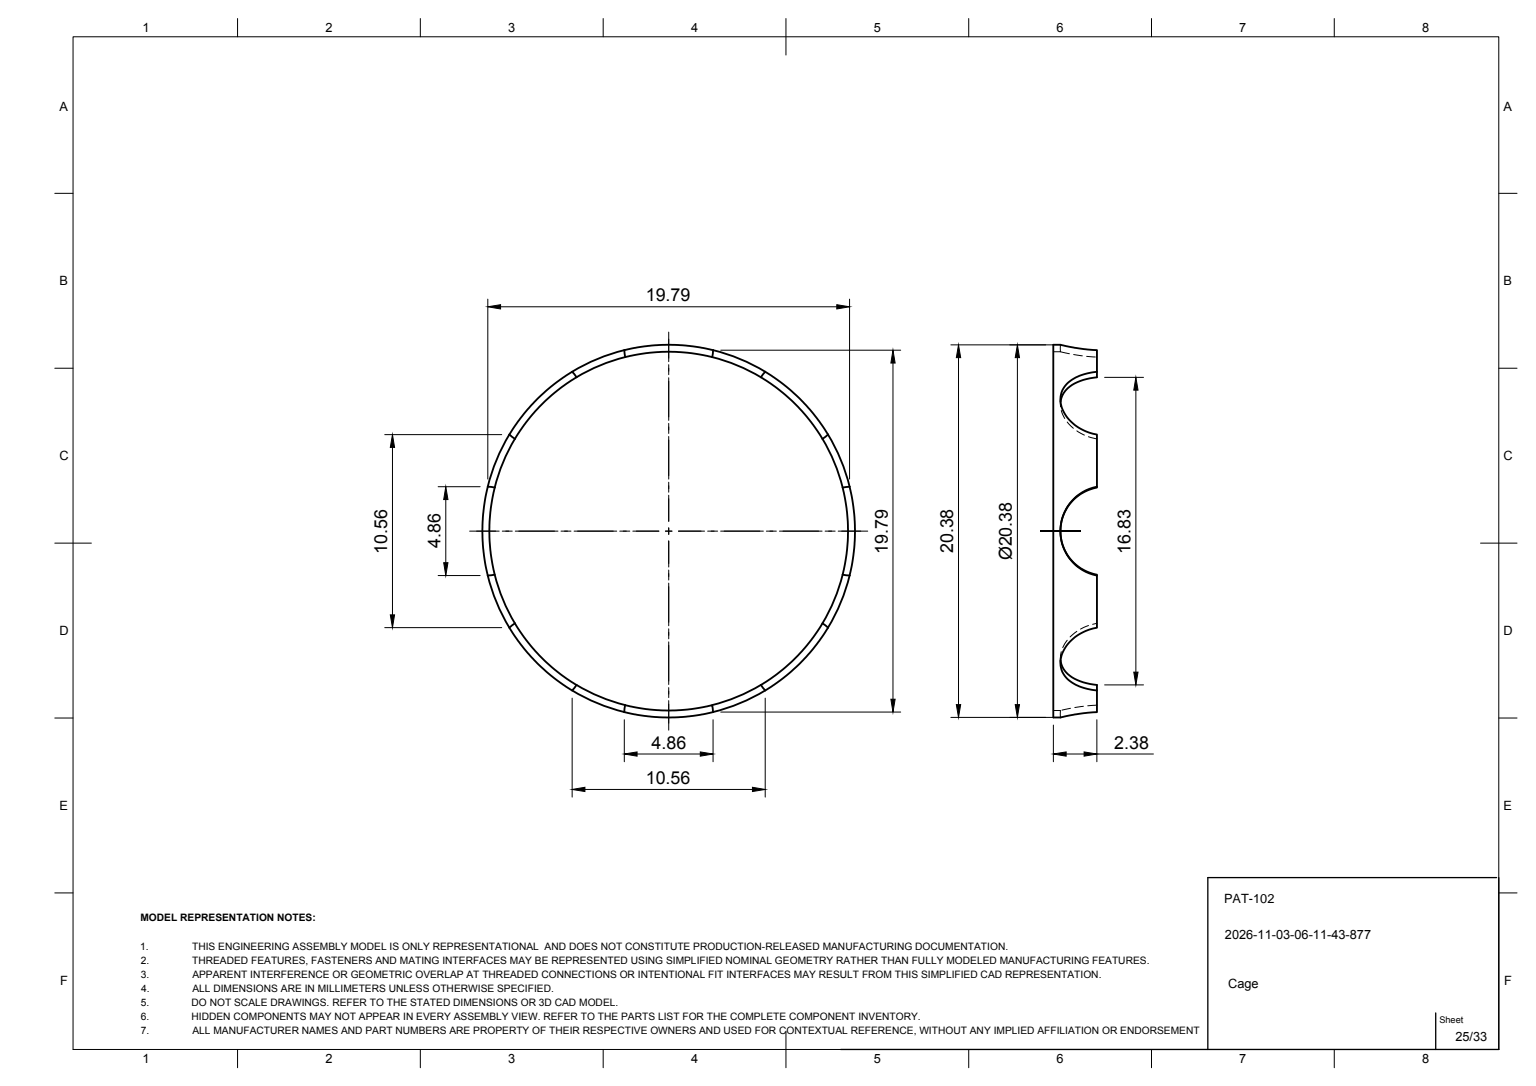
ISO-10303-21;
HEADER;
/* Generated by software containing ST-Developer
 * from STEP Tools, Inc. (www.steptools.com) 
 */

FILE_DESCRIPTION(
/* description */ ('Swing-away clamp arm'),
/* implementation_level */ '2;1');

FILE_NAME(
/* name */ 'Cage.step',
/* time_stamp */ '2026-10-28T03:26:03-07:00',
/* author */ (''),
/* organization */ (''),
/* preprocessor_version */ 'ST-DEVELOPER v20.2',
/* originating_system */ 'Autodesk Translation Framework v15.17.0.0',
/* authorisation */ '');

FILE_SCHEMA (('AUTOMOTIVE_DESIGN { 1 0 10303 214 3 1 1 }'));
ENDSEC;

DATA;
#10=MECHANICAL_DESIGN_GEOMETRIC_PRESENTATION_REPRESENTATION('',(#317),#10627);
#19=SPHERICAL_SURFACE('',#5638,0.247676);
#20=SPHERICAL_SURFACE('',#5654,0.247676);
#21=SPHERICAL_SURFACE('',#5659,0.247676);
#22=SPHERICAL_SURFACE('',#5664,0.247676);
#23=SPHERICAL_SURFACE('',#5669,0.247676);
#24=SPHERICAL_SURFACE('',#5674,0.247676);
#25=SPHERICAL_SURFACE('',#5679,0.247676);
#26=SPHERICAL_SURFACE('',#5687,0.247676);
#222=B_SPLINE_CURVE_WITH_KNOTS('',3,(#9779,#9780,#9781,#9782,#9783,#9784,
#9785,#9786,#9787,#9788,#9789,#9790,#9791,#9792,#9793,#9794,#9795,#9796,
#9797,#9798,#9799,#9800),.UNSPECIFIED.,.F.,.F.,(4,2,2,2,2,2,2,2,2,2,4),
(0.0473477652366656,0.126350602536658,0.189525903804987,0.252701205073317,
0.313298422430275,0.373895639787233,0.434492857144191,0.495090074501149,
0.558265375769478,0.621440677037807,0.7004435143378),.UNSPECIFIED.);
#223=B_SPLINE_CURVE_WITH_KNOTS('',3,(#9804,#9805,#9806,#9807,#9808,#9809,
#9810,#9811,#9812,#9813,#9814,#9815,#9816,#9817,#9818,#9819,#9820,#9821,
#9822,#9823,#9824,#9825),.UNSPECIFIED.,.F.,.F.,(4,2,2,2,2,2,2,2,2,2,4),
(0.0464897534940957,0.0852567806515119,0.170513561303024,0.246687263103517,
0.308657850341199,0.370628437578881,0.432599024816563,0.494569612054245,
0.570743313854739,0.656000094506251,0.694767121663666),.UNSPECIFIED.);
#224=B_SPLINE_CURVE_WITH_KNOTS('',3,(#9831,#9832,#9833,#9834,#9835,#9836,
#9837,#9838,#9839,#9840,#9841,#9842,#9843,#9844,#9845,#9846,#9847,#9848,
#9849,#9850,#9851,#9852),.UNSPECIFIED.,.F.,.F.,(4,2,2,2,2,2,2,2,2,2,4),
(0.0464897534940957,0.0852567806515118,0.170513561303024,0.246687263103517,
0.308657850341199,0.370628437578881,0.432599024816563,0.494569612054245,
0.570743313854738,0.65600009450625,0.694767121663666),.UNSPECIFIED.);
#225=B_SPLINE_CURVE_WITH_KNOTS('',3,(#9856,#9857,#9858,#9859,#9860,#9861,
#9862,#9863,#9864,#9865,#9866,#9867,#9868,#9869,#9870,#9871,#9872,#9873,
#9874,#9875,#9876,#9877),.UNSPECIFIED.,.F.,.F.,(4,2,2,2,2,2,2,2,2,2,4),
(0.0464897534940957,0.0852567806515119,0.170513561303024,0.246687263103517,
0.308657850341199,0.370628437578881,0.432599024816563,0.494569612054245,
0.570743313854739,0.656000094506251,0.694767121663666),.UNSPECIFIED.);
#226=B_SPLINE_CURVE_WITH_KNOTS('',3,(#9881,#9882,#9883,#9884,#9885,#9886,
#9887,#9888,#9889,#9890,#9891,#9892),.UNSPECIFIED.,.F.,.F.,(4,2,2,2,2,4),
(0.0464897534940957,0.0852567806515119,0.170513561303024,0.246687263103517,
0.308657850341199,0.370628437578881),.UNSPECIFIED.);
#227=B_SPLINE_CURVE_WITH_KNOTS('',3,(#9897,#9898,#9899,#9900,#9901,#9902,
#9903,#9904,#9905,#9906,#9907,#9908),.UNSPECIFIED.,.F.,.F.,(4,2,2,2,2,4),
(0.370628437578881,0.432599024816563,0.494569612054245,0.570743313854738,
0.65600009450625,0.694767121663666),.UNSPECIFIED.);
#228=B_SPLINE_CURVE_WITH_KNOTS('',3,(#9912,#9913,#9914,#9915,#9916,#9917,
#9918,#9919,#9920,#9921,#9922,#9923,#9924,#9925,#9926,#9927,#9928,#9929,
#9930,#9931,#9932,#9933),.UNSPECIFIED.,.F.,.F.,(4,2,2,2,2,2,2,2,2,2,4),
(0.0464897534940957,0.0852567806515121,0.170513561303024,0.246687263103518,
0.308657850341199,0.370628437578881,0.432599024816563,0.494569612054245,
0.570743313854738,0.65600009450625,0.694767121663666),.UNSPECIFIED.);
#229=B_SPLINE_CURVE_WITH_KNOTS('',3,(#9937,#9938,#9939,#9940,#9941,#9942,
#9943,#9944,#9945,#9946,#9947,#9948,#9949,#9950,#9951,#9952,#9953,#9954,
#9955,#9956,#9957,#9958),.UNSPECIFIED.,.F.,.F.,(4,2,2,2,2,2,2,2,2,2,4),
(0.0464897534940957,0.0852567806515119,0.170513561303024,0.246687263103517,
0.308657850341199,0.370628437578881,0.432599024816563,0.494569612054245,
0.570743313854738,0.65600009450625,0.694767121663667),.UNSPECIFIED.);
#230=B_SPLINE_CURVE_WITH_KNOTS('',3,(#9962,#9963,#9964,#9965,#9966,#9967,
#9968,#9969,#9970,#9971,#9972,#9973,#9974,#9975,#9976,#9977,#9978,#9979,
#9980,#9981,#9982,#9983),.UNSPECIFIED.,.F.,.F.,(4,2,2,2,2,2,2,2,2,2,4),
(0.0464897534940957,0.0852567806515119,0.170513561303024,0.246687263103517,
0.308657850341199,0.370628437578881,0.432599024816563,0.494569612054245,
0.570743313854738,0.65600009450625,0.694767121663666),.UNSPECIFIED.);
#231=B_SPLINE_CURVE_WITH_KNOTS('',3,(#9987,#9988,#9989,#9990,#9991,#9992,
#9993,#9994,#9995,#9996,#9997,#9998,#9999,#10000,#10001,#10002,#10003,#10004,
#10005,#10006,#10007,#10008),.UNSPECIFIED.,.F.,.F.,(4,2,2,2,2,2,2,2,2,2,
4),(0.0464897534940957,0.0852567806515119,0.170513561303024,0.246687263103517,
0.308657850341199,0.370628437578881,0.432599024816563,0.494569612054245,
0.570743313854739,0.656000094506251,0.694767121663667),.UNSPECIFIED.);
#232=B_SPLINE_CURVE_WITH_KNOTS('',3,(#10016,#10017,#10018,#10019,#10020,
#10021,#10022,#10023,#10024,#10025,#10026,#10027,#10028,#10029,#10030,#10031,
#10032,#10033,#10034,#10035,#10036,#10037),.UNSPECIFIED.,.F.,.F.,(4,2,2,
2,2,2,2,2,2,2,4),(0.0473477652366656,0.126350602536658,0.189525903804987,
0.252701205073316,0.313298422430274,0.373895639787232,0.434492857144191,
0.495090074501149,0.558265375769478,0.621440677037807,0.7004435143378),
 .UNSPECIFIED.);
#233=B_SPLINE_CURVE_WITH_KNOTS('',3,(#10045,#10046,#10047,#10048,#10049,
#10050,#10051,#10052,#10053,#10054,#10055,#10056,#10057,#10058,#10059,#10060,
#10061,#10062,#10063,#10064,#10065,#10066),.UNSPECIFIED.,.F.,.F.,(4,2,2,
2,2,2,2,2,2,2,4),(0.0473477652366656,0.126350602536658,0.189525903804987,
0.252701205073317,0.313298422430275,0.373895639787233,0.434492857144191,
0.495090074501149,0.558265375769478,0.621440677037807,0.7004435143378),
 .UNSPECIFIED.);
#234=B_SPLINE_CURVE_WITH_KNOTS('',3,(#10075,#10076,#10077,#10078,#10079,
#10080,#10081,#10082,#10083,#10084,#10085,#10086),.UNSPECIFIED.,.F.,.F.,
(4,2,2,2,2,4),(0.0473477652366656,0.126350602536658,0.189525903804987,0.252701205073316,
0.313298422430275,0.373895639787233),.UNSPECIFIED.);
#235=B_SPLINE_CURVE_WITH_KNOTS('',3,(#10088,#10089,#10090,#10091,#10092,
#10093,#10094,#10095,#10096,#10097,#10098,#10099),.UNSPECIFIED.,.F.,.F.,
(4,2,2,2,2,4),(0.373895639787233,0.434492857144191,0.495090074501149,0.558265375769478,
0.621440677037807,0.7004435143378),.UNSPECIFIED.);
#236=B_SPLINE_CURVE_WITH_KNOTS('',3,(#10106,#10107,#10108,#10109,#10110,
#10111,#10112,#10113,#10114,#10115,#10116,#10117,#10118,#10119,#10120,#10121,
#10122,#10123,#10124,#10125,#10126,#10127),.UNSPECIFIED.,.F.,.F.,(4,2,2,
2,2,2,2,2,2,2,4),(0.0473477652366656,0.126350602536658,0.189525903804987,
0.252701205073316,0.313298422430275,0.373895639787233,0.434492857144191,
0.495090074501149,0.558265375769478,0.621440677037807,0.7004435143378),
 .UNSPECIFIED.);
#237=B_SPLINE_CURVE_WITH_KNOTS('',3,(#10135,#10136,#10137,#10138,#10139,
#10140,#10141,#10142,#10143,#10144,#10145,#10146,#10147,#10148,#10149,#10150,
#10151,#10152,#10153,#10154,#10155,#10156),.UNSPECIFIED.,.F.,.F.,(4,2,2,
2,2,2,2,2,2,2,4),(0.0473477652366656,0.126350602536658,0.189525903804987,
0.252701205073317,0.313298422430275,0.373895639787233,0.434492857144191,
0.495090074501149,0.558265375769478,0.621440677037807,0.7004435143378),
 .UNSPECIFIED.);
#238=B_SPLINE_CURVE_WITH_KNOTS('',3,(#10164,#10165,#10166,#10167,#10168,
#10169,#10170,#10171,#10172,#10173,#10174,#10175,#10176,#10177,#10178,#10179,
#10180,#10181,#10182,#10183,#10184,#10185),.UNSPECIFIED.,.F.,.F.,(4,2,2,
2,2,2,2,2,2,2,4),(0.0473477652366656,0.126350602536658,0.189525903804987,
0.252701205073316,0.313298422430275,0.373895639787233,0.434492857144191,
0.495090074501149,0.558265375769478,0.621440677037807,0.7004435143378),
 .UNSPECIFIED.);
#239=B_SPLINE_CURVE_WITH_KNOTS('',3,(#10194,#10195,#10196,#10197,#10198,
#10199,#10200,#10201,#10202,#10203,#10204,#10205,#10206,#10207,#10208,#10209,
#10210,#10211,#10212,#10213,#10214,#10215),.UNSPECIFIED.,.F.,.F.,(4,2,2,
2,2,2,2,2,2,2,4),(0.0473477652366656,0.126350602536658,0.189525903804987,
0.252701205073317,0.313298422430275,0.373895639787233,0.434492857144191,
0.495090074501149,0.558265375769478,0.621440677037807,0.7004435143378),
 .UNSPECIFIED.);
#258=SHAPE_REPRESENTATION_RELATIONSHIP('SRR','None',#10758,#284);
#284=ADVANCED_BREP_SHAPE_REPRESENTATION('',(#350),#10617);
#317=STYLED_ITEM('',(#10965),#350);
#350=MANIFOLD_SOLID_BREP('Continuous crown cage',#4924);
#436=FACE_BOUND('',#1250,.T.);
#582=PLANE('',#5651);
#583=PLANE('',#5656);
#584=PLANE('',#5661);
#585=PLANE('',#5666);
#586=PLANE('',#5671);
#587=PLANE('',#5676);
#588=PLANE('',#5685);
#589=PLANE('',#5689);
#590=PLANE('',#5690);
#847=FACE_OUTER_BOUND('',#1232,.T.);
#848=FACE_OUTER_BOUND('',#1233,.T.);
#849=FACE_OUTER_BOUND('',#1234,.T.);
#850=FACE_OUTER_BOUND('',#1235,.T.);
#851=FACE_OUTER_BOUND('',#1236,.T.);
#852=FACE_OUTER_BOUND('',#1237,.T.);
#853=FACE_OUTER_BOUND('',#1238,.T.);
#854=FACE_OUTER_BOUND('',#1239,.T.);
#855=FACE_OUTER_BOUND('',#1240,.T.);
#856=FACE_OUTER_BOUND('',#1241,.T.);
#857=FACE_OUTER_BOUND('',#1242,.T.);
#858=FACE_OUTER_BOUND('',#1243,.T.);
#859=FACE_OUTER_BOUND('',#1244,.T.);
#860=FACE_OUTER_BOUND('',#1245,.T.);
#861=FACE_OUTER_BOUND('',#1246,.T.);
#862=FACE_OUTER_BOUND('',#1247,.T.);
#863=FACE_OUTER_BOUND('',#1248,.T.);
#864=FACE_OUTER_BOUND('',#1249,.T.);
#865=FACE_OUTER_BOUND('',#1251,.T.);
#1232=EDGE_LOOP('',(#4121,#4122,#4123,#4124));
#1233=EDGE_LOOP('',(#4125,#4126,#4127,#4128,#4129,#4130,#4131,#4132,#4133,
#4134,#4135,#4136,#4137,#4138,#4139,#4140,#4141,#4142,#4143,#4144));
#1234=EDGE_LOOP('',(#4145,#4146,#4147,#4148));
#1235=EDGE_LOOP('',(#4149,#4150,#4151,#4152));
#1236=EDGE_LOOP('',(#4153,#4154,#4155,#4156));
#1237=EDGE_LOOP('',(#4157,#4158,#4159,#4160));
#1238=EDGE_LOOP('',(#4161,#4162,#4163,#4164));
#1239=EDGE_LOOP('',(#4165,#4166,#4167,#4168,#4169,#4170));
#1240=EDGE_LOOP('',(#4171,#4172,#4173,#4174));
#1241=EDGE_LOOP('',(#4175,#4176,#4177,#4178));
#1242=EDGE_LOOP('',(#4179,#4180,#4181,#4182));
#1243=EDGE_LOOP('',(#4183,#4184,#4185,#4186));
#1244=EDGE_LOOP('',(#4187,#4188,#4189,#4190));
#1245=EDGE_LOOP('',(#4191,#4192,#4193,#4194));
#1246=EDGE_LOOP('',(#4195,#4196,#4197,#4198,#4199,#4200,#4201,#4202,#4203,
#4204,#4205,#4206,#4207,#4208,#4209,#4210,#4211,#4212,#4213,#4214));
#1247=EDGE_LOOP('',(#4215,#4216,#4217,#4218));
#1248=EDGE_LOOP('',(#4219,#4220,#4221,#4222));
#1249=EDGE_LOOP('',(#4223));
#1250=EDGE_LOOP('',(#4224));
#1251=EDGE_LOOP('',(#4225,#4226,#4227,#4228));
#1596=LINE('',#9894,#1918);
#1597=LINE('',#10190,#1919);
#1918=VECTOR('',#6959,1.019052);
#1919=VECTOR('',#7036,0.980948);
#2169=CIRCLE('',#5639,0.243053047864041);
#2170=CIRCLE('',#5640,0.243053047864041);
#2171=CIRCLE('',#5642,1.019052);
#2172=CIRCLE('',#5643,1.019052);
#2173=CIRCLE('',#5644,1.019052);
#2174=CIRCLE('',#5645,1.019052);
#2175=CIRCLE('',#5646,1.019052);
#2176=CIRCLE('',#5647,1.019052);
#2177=CIRCLE('',#5648,1.019052);
#2178=CIRCLE('',#5649,1.019052);
#2179=CIRCLE('',#5650,1.019052);
#2180=CIRCLE('',#5652,0.980948);
#2181=CIRCLE('',#5653,0.243053047864041);
#2182=CIRCLE('',#5655,0.243053047864041);
#2183=CIRCLE('',#5657,0.980948);
#2184=CIRCLE('',#5658,0.243053047864041);
#2185=CIRCLE('',#5660,0.243053047864041);
#2186=CIRCLE('',#5662,0.980948);
#2187=CIRCLE('',#5663,0.243053047864041);
#2188=CIRCLE('',#5665,0.243053047864041);
#2189=CIRCLE('',#5667,0.980948);
#2190=CIRCLE('',#5668,0.243053047864041);
#2191=CIRCLE('',#5670,0.243053047864041);
#2192=CIRCLE('',#5672,0.980948);
#2193=CIRCLE('',#5673,0.243053047864041);
#2194=CIRCLE('',#5675,0.243053047864041);
#2195=CIRCLE('',#5677,0.980948);
#2196=CIRCLE('',#5678,0.243053047864041);
#2197=CIRCLE('',#5680,0.243053047864041);
#2198=CIRCLE('',#5682,0.980948);
#2199=CIRCLE('',#5683,0.980948);
#2200=CIRCLE('',#5684,0.980948);
#2201=CIRCLE('',#5686,0.243053047864041);
#2202=CIRCLE('',#5688,0.243053047864041);
#2550=VERTEX_POINT('',#9777);
#2551=VERTEX_POINT('',#9778);
#2552=VERTEX_POINT('',#9801);
#2553=VERTEX_POINT('',#9803);
#2554=VERTEX_POINT('',#9828);
#2555=VERTEX_POINT('',#9830);
#2556=VERTEX_POINT('',#9853);
#2557=VERTEX_POINT('',#9855);
#2558=VERTEX_POINT('',#9878);
#2559=VERTEX_POINT('',#9880);
#2560=VERTEX_POINT('',#9893);
#2561=VERTEX_POINT('',#9896);
#2562=VERTEX_POINT('',#9909);
#2563=VERTEX_POINT('',#9911);
#2564=VERTEX_POINT('',#9934);
#2565=VERTEX_POINT('',#9936);
#2566=VERTEX_POINT('',#9959);
#2567=VERTEX_POINT('',#9961);
#2568=VERTEX_POINT('',#9984);
#2569=VERTEX_POINT('',#9986);
#2570=VERTEX_POINT('',#10011);
#2571=VERTEX_POINT('',#10015);
#2572=VERTEX_POINT('',#10040);
#2573=VERTEX_POINT('',#10044);
#2574=VERTEX_POINT('',#10069);
#2575=VERTEX_POINT('',#10073);
#2576=VERTEX_POINT('',#10074);
#2577=VERTEX_POINT('',#10101);
#2578=VERTEX_POINT('',#10105);
#2579=VERTEX_POINT('',#10130);
#2580=VERTEX_POINT('',#10134);
#2581=VERTEX_POINT('',#10159);
#2582=VERTEX_POINT('',#10163);
#2583=VERTEX_POINT('',#10188);
#2584=VERTEX_POINT('',#10191);
#2585=VERTEX_POINT('',#10193);
#3093=EDGE_CURVE('',#2550,#2551,#222,.T.);
#3094=EDGE_CURVE('',#2552,#2550,#2169,.T.);
#3095=EDGE_CURVE('',#2553,#2552,#223,.T.);
#3096=EDGE_CURVE('',#2551,#2553,#2170,.T.);
#3097=EDGE_CURVE('',#2554,#2552,#2171,.T.);
#3098=EDGE_CURVE('',#2554,#2555,#224,.T.);
#3099=EDGE_CURVE('',#2556,#2555,#2172,.T.);
#3100=EDGE_CURVE('',#2556,#2557,#225,.T.);
#3101=EDGE_CURVE('',#2558,#2557,#2173,.T.);
#3102=EDGE_CURVE('',#2558,#2559,#226,.T.);
#3103=EDGE_CURVE('',#2559,#2560,#1596,.T.);
#3104=EDGE_CURVE('',#2560,#2560,#2174,.T.);
#3105=EDGE_CURVE('',#2559,#2561,#227,.T.);
#3106=EDGE_CURVE('',#2562,#2561,#2175,.T.);
#3107=EDGE_CURVE('',#2562,#2563,#228,.T.);
#3108=EDGE_CURVE('',#2564,#2563,#2176,.T.);
#3109=EDGE_CURVE('',#2564,#2565,#229,.T.);
#3110=EDGE_CURVE('',#2566,#2565,#2177,.T.);
#3111=EDGE_CURVE('',#2566,#2567,#230,.T.);
#3112=EDGE_CURVE('',#2568,#2567,#2178,.T.);
#3113=EDGE_CURVE('',#2568,#2569,#231,.T.);
#3114=EDGE_CURVE('',#2553,#2569,#2179,.T.);
#3115=EDGE_CURVE('',#2550,#2570,#2180,.T.);
#3116=EDGE_CURVE('',#2570,#2554,#2181,.T.);
#3117=EDGE_CURVE('',#2571,#2570,#232,.T.);
#3118=EDGE_CURVE('',#2555,#2571,#2182,.T.);
#3119=EDGE_CURVE('',#2571,#2572,#2183,.T.);
#3120=EDGE_CURVE('',#2572,#2556,#2184,.T.);
#3121=EDGE_CURVE('',#2573,#2572,#233,.T.);
#3122=EDGE_CURVE('',#2557,#2573,#2185,.T.);
#3123=EDGE_CURVE('',#2573,#2574,#2186,.T.);
#3124=EDGE_CURVE('',#2574,#2558,#2187,.T.);
#3125=EDGE_CURVE('',#2575,#2576,#234,.T.);
#3126=EDGE_CURVE('',#2561,#2575,#2188,.T.);
#3127=EDGE_CURVE('',#2576,#2574,#235,.T.);
#3128=EDGE_CURVE('',#2575,#2577,#2189,.T.);
#3129=EDGE_CURVE('',#2577,#2562,#2190,.T.);
#3130=EDGE_CURVE('',#2578,#2577,#236,.T.);
#3131=EDGE_CURVE('',#2563,#2578,#2191,.T.);
#3132=EDGE_CURVE('',#2578,#2579,#2192,.T.);
#3133=EDGE_CURVE('',#2579,#2564,#2193,.T.);
#3134=EDGE_CURVE('',#2580,#2579,#237,.T.);
#3135=EDGE_CURVE('',#2565,#2580,#2194,.T.);
#3136=EDGE_CURVE('',#2580,#2581,#2195,.T.);
#3137=EDGE_CURVE('',#2581,#2566,#2196,.T.);
#3138=EDGE_CURVE('',#2582,#2581,#238,.T.);
#3139=EDGE_CURVE('',#2567,#2582,#2197,.T.);
#3140=EDGE_CURVE('',#2583,#2583,#2198,.T.);
#3141=EDGE_CURVE('',#2583,#2576,#1597,.T.);
#3142=EDGE_CURVE('',#2584,#2551,#2199,.T.);
#3143=EDGE_CURVE('',#2584,#2585,#239,.T.);
#3144=EDGE_CURVE('',#2582,#2585,#2200,.T.);
#3145=EDGE_CURVE('',#2569,#2584,#2201,.T.);
#3146=EDGE_CURVE('',#2585,#2568,#2202,.T.);
#4121=ORIENTED_EDGE('',*,*,#3093,.F.);
#4122=ORIENTED_EDGE('',*,*,#3094,.F.);
#4123=ORIENTED_EDGE('',*,*,#3095,.F.);
#4124=ORIENTED_EDGE('',*,*,#3096,.F.);
#4125=ORIENTED_EDGE('',*,*,#3095,.T.);
#4126=ORIENTED_EDGE('',*,*,#3097,.F.);
#4127=ORIENTED_EDGE('',*,*,#3098,.T.);
#4128=ORIENTED_EDGE('',*,*,#3099,.F.);
#4129=ORIENTED_EDGE('',*,*,#3100,.T.);
#4130=ORIENTED_EDGE('',*,*,#3101,.F.);
#4131=ORIENTED_EDGE('',*,*,#3102,.T.);
#4132=ORIENTED_EDGE('',*,*,#3103,.T.);
#4133=ORIENTED_EDGE('',*,*,#3104,.F.);
#4134=ORIENTED_EDGE('',*,*,#3103,.F.);
#4135=ORIENTED_EDGE('',*,*,#3105,.T.);
#4136=ORIENTED_EDGE('',*,*,#3106,.F.);
#4137=ORIENTED_EDGE('',*,*,#3107,.T.);
#4138=ORIENTED_EDGE('',*,*,#3108,.F.);
#4139=ORIENTED_EDGE('',*,*,#3109,.T.);
#4140=ORIENTED_EDGE('',*,*,#3110,.F.);
#4141=ORIENTED_EDGE('',*,*,#3111,.T.);
#4142=ORIENTED_EDGE('',*,*,#3112,.F.);
#4143=ORIENTED_EDGE('',*,*,#3113,.T.);
#4144=ORIENTED_EDGE('',*,*,#3114,.F.);
#4145=ORIENTED_EDGE('',*,*,#3094,.T.);
#4146=ORIENTED_EDGE('',*,*,#3115,.T.);
#4147=ORIENTED_EDGE('',*,*,#3116,.T.);
#4148=ORIENTED_EDGE('',*,*,#3097,.T.);
#4149=ORIENTED_EDGE('',*,*,#3117,.F.);
#4150=ORIENTED_EDGE('',*,*,#3118,.F.);
#4151=ORIENTED_EDGE('',*,*,#3098,.F.);
#4152=ORIENTED_EDGE('',*,*,#3116,.F.);
#4153=ORIENTED_EDGE('',*,*,#3118,.T.);
#4154=ORIENTED_EDGE('',*,*,#3119,.T.);
#4155=ORIENTED_EDGE('',*,*,#3120,.T.);
#4156=ORIENTED_EDGE('',*,*,#3099,.T.);
#4157=ORIENTED_EDGE('',*,*,#3121,.F.);
#4158=ORIENTED_EDGE('',*,*,#3122,.F.);
#4159=ORIENTED_EDGE('',*,*,#3100,.F.);
#4160=ORIENTED_EDGE('',*,*,#3120,.F.);
#4161=ORIENTED_EDGE('',*,*,#3122,.T.);
#4162=ORIENTED_EDGE('',*,*,#3123,.T.);
#4163=ORIENTED_EDGE('',*,*,#3124,.T.);
#4164=ORIENTED_EDGE('',*,*,#3101,.T.);
#4165=ORIENTED_EDGE('',*,*,#3125,.F.);
#4166=ORIENTED_EDGE('',*,*,#3126,.F.);
#4167=ORIENTED_EDGE('',*,*,#3105,.F.);
#4168=ORIENTED_EDGE('',*,*,#3102,.F.);
#4169=ORIENTED_EDGE('',*,*,#3124,.F.);
#4170=ORIENTED_EDGE('',*,*,#3127,.F.);
#4171=ORIENTED_EDGE('',*,*,#3126,.T.);
#4172=ORIENTED_EDGE('',*,*,#3128,.T.);
#4173=ORIENTED_EDGE('',*,*,#3129,.T.);
#4174=ORIENTED_EDGE('',*,*,#3106,.T.);
#4175=ORIENTED_EDGE('',*,*,#3130,.F.);
#4176=ORIENTED_EDGE('',*,*,#3131,.F.);
#4177=ORIENTED_EDGE('',*,*,#3107,.F.);
#4178=ORIENTED_EDGE('',*,*,#3129,.F.);
#4179=ORIENTED_EDGE('',*,*,#3131,.T.);
#4180=ORIENTED_EDGE('',*,*,#3132,.T.);
#4181=ORIENTED_EDGE('',*,*,#3133,.T.);
#4182=ORIENTED_EDGE('',*,*,#3108,.T.);
#4183=ORIENTED_EDGE('',*,*,#3134,.F.);
#4184=ORIENTED_EDGE('',*,*,#3135,.F.);
#4185=ORIENTED_EDGE('',*,*,#3109,.F.);
#4186=ORIENTED_EDGE('',*,*,#3133,.F.);
#4187=ORIENTED_EDGE('',*,*,#3135,.T.);
#4188=ORIENTED_EDGE('',*,*,#3136,.T.);
#4189=ORIENTED_EDGE('',*,*,#3137,.T.);
#4190=ORIENTED_EDGE('',*,*,#3110,.T.);
#4191=ORIENTED_EDGE('',*,*,#3111,.F.);
#4192=ORIENTED_EDGE('',*,*,#3137,.F.);
#4193=ORIENTED_EDGE('',*,*,#3138,.F.);
#4194=ORIENTED_EDGE('',*,*,#3139,.F.);
#4195=ORIENTED_EDGE('',*,*,#3140,.F.);
#4196=ORIENTED_EDGE('',*,*,#3141,.T.);
#4197=ORIENTED_EDGE('',*,*,#3127,.T.);
#4198=ORIENTED_EDGE('',*,*,#3123,.F.);
#4199=ORIENTED_EDGE('',*,*,#3121,.T.);
#4200=ORIENTED_EDGE('',*,*,#3119,.F.);
#4201=ORIENTED_EDGE('',*,*,#3117,.T.);
#4202=ORIENTED_EDGE('',*,*,#3115,.F.);
#4203=ORIENTED_EDGE('',*,*,#3093,.T.);
#4204=ORIENTED_EDGE('',*,*,#3142,.F.);
#4205=ORIENTED_EDGE('',*,*,#3143,.T.);
#4206=ORIENTED_EDGE('',*,*,#3144,.F.);
#4207=ORIENTED_EDGE('',*,*,#3138,.T.);
#4208=ORIENTED_EDGE('',*,*,#3136,.F.);
#4209=ORIENTED_EDGE('',*,*,#3134,.T.);
#4210=ORIENTED_EDGE('',*,*,#3132,.F.);
#4211=ORIENTED_EDGE('',*,*,#3130,.T.);
#4212=ORIENTED_EDGE('',*,*,#3128,.F.);
#4213=ORIENTED_EDGE('',*,*,#3125,.T.);
#4214=ORIENTED_EDGE('',*,*,#3141,.F.);
#4215=ORIENTED_EDGE('',*,*,#3096,.T.);
#4216=ORIENTED_EDGE('',*,*,#3114,.T.);
#4217=ORIENTED_EDGE('',*,*,#3145,.T.);
#4218=ORIENTED_EDGE('',*,*,#3142,.T.);
#4219=ORIENTED_EDGE('',*,*,#3113,.F.);
#4220=ORIENTED_EDGE('',*,*,#3146,.F.);
#4221=ORIENTED_EDGE('',*,*,#3143,.F.);
#4222=ORIENTED_EDGE('',*,*,#3145,.F.);
#4223=ORIENTED_EDGE('',*,*,#3104,.T.);
#4224=ORIENTED_EDGE('',*,*,#3140,.T.);
#4225=ORIENTED_EDGE('',*,*,#3139,.T.);
#4226=ORIENTED_EDGE('',*,*,#3144,.T.);
#4227=ORIENTED_EDGE('',*,*,#3146,.T.);
#4228=ORIENTED_EDGE('',*,*,#3112,.T.);
#4565=CYLINDRICAL_SURFACE('',#5641,1.019052);
#4566=CYLINDRICAL_SURFACE('',#5681,0.980948);
#4802=ADVANCED_FACE('',(#847),#19,.F.);
#4803=ADVANCED_FACE('',(#848),#4565,.T.);
#4804=ADVANCED_FACE('',(#849),#582,.T.);
#4805=ADVANCED_FACE('',(#850),#20,.F.);
#4806=ADVANCED_FACE('',(#851),#583,.T.);
#4807=ADVANCED_FACE('',(#852),#21,.F.);
#4808=ADVANCED_FACE('',(#853),#584,.T.);
#4809=ADVANCED_FACE('',(#854),#22,.F.);
#4810=ADVANCED_FACE('',(#855),#585,.T.);
#4811=ADVANCED_FACE('',(#856),#23,.F.);
#4812=ADVANCED_FACE('',(#857),#586,.T.);
#4813=ADVANCED_FACE('',(#858),#24,.F.);
#4814=ADVANCED_FACE('',(#859),#587,.T.);
#4815=ADVANCED_FACE('',(#860),#25,.F.);
#4816=ADVANCED_FACE('',(#861),#4566,.F.);
#4817=ADVANCED_FACE('',(#862),#588,.T.);
#4818=ADVANCED_FACE('',(#863),#26,.F.);
#4819=ADVANCED_FACE('',(#864,#436),#589,.T.);
#4820=ADVANCED_FACE('',(#865),#590,.T.);
#4924=CLOSED_SHELL('',(#4802,#4803,#4804,#4805,#4806,#4807,#4808,#4809,
#4810,#4811,#4812,#4813,#4814,#4815,#4816,#4817,#4818,#4819,#4820));
#5637=AXIS2_PLACEMENT_3D('',#9775,#6943,#6944);
#5638=AXIS2_PLACEMENT_3D('',#9776,#6945,#6946);
#5639=AXIS2_PLACEMENT_3D('',#9802,#6947,#6948);
#5640=AXIS2_PLACEMENT_3D('',#9826,#6949,#6950);
#5641=AXIS2_PLACEMENT_3D('',#9827,#6951,#6952);
#5642=AXIS2_PLACEMENT_3D('',#9829,#6953,#6954);
#5643=AXIS2_PLACEMENT_3D('',#9854,#6955,#6956);
#5644=AXIS2_PLACEMENT_3D('',#9879,#6957,#6958);
#5645=AXIS2_PLACEMENT_3D('',#9895,#6960,#6961);
#5646=AXIS2_PLACEMENT_3D('',#9910,#6962,#6963);
#5647=AXIS2_PLACEMENT_3D('',#9935,#6964,#6965);
#5648=AXIS2_PLACEMENT_3D('',#9960,#6966,#6967);
#5649=AXIS2_PLACEMENT_3D('',#9985,#6968,#6969);
#5650=AXIS2_PLACEMENT_3D('',#10009,#6970,#6971);
#5651=AXIS2_PLACEMENT_3D('',#10010,#6972,#6973);
#5652=AXIS2_PLACEMENT_3D('',#10012,#6974,#6975);
#5653=AXIS2_PLACEMENT_3D('',#10013,#6976,#6977);
#5654=AXIS2_PLACEMENT_3D('',#10014,#6978,#6979);
#5655=AXIS2_PLACEMENT_3D('',#10038,#6980,#6981);
#5656=AXIS2_PLACEMENT_3D('',#10039,#6982,#6983);
#5657=AXIS2_PLACEMENT_3D('',#10041,#6984,#6985);
#5658=AXIS2_PLACEMENT_3D('',#10042,#6986,#6987);
#5659=AXIS2_PLACEMENT_3D('',#10043,#6988,#6989);
#5660=AXIS2_PLACEMENT_3D('',#10067,#6990,#6991);
#5661=AXIS2_PLACEMENT_3D('',#10068,#6992,#6993);
#5662=AXIS2_PLACEMENT_3D('',#10070,#6994,#6995);
#5663=AXIS2_PLACEMENT_3D('',#10071,#6996,#6997);
#5664=AXIS2_PLACEMENT_3D('',#10072,#6998,#6999);
#5665=AXIS2_PLACEMENT_3D('',#10087,#7000,#7001);
#5666=AXIS2_PLACEMENT_3D('',#10100,#7002,#7003);
#5667=AXIS2_PLACEMENT_3D('',#10102,#7004,#7005);
#5668=AXIS2_PLACEMENT_3D('',#10103,#7006,#7007);
#5669=AXIS2_PLACEMENT_3D('',#10104,#7008,#7009);
#5670=AXIS2_PLACEMENT_3D('',#10128,#7010,#7011);
#5671=AXIS2_PLACEMENT_3D('',#10129,#7012,#7013);
#5672=AXIS2_PLACEMENT_3D('',#10131,#7014,#7015);
#5673=AXIS2_PLACEMENT_3D('',#10132,#7016,#7017);
#5674=AXIS2_PLACEMENT_3D('',#10133,#7018,#7019);
#5675=AXIS2_PLACEMENT_3D('',#10157,#7020,#7021);
#5676=AXIS2_PLACEMENT_3D('',#10158,#7022,#7023);
#5677=AXIS2_PLACEMENT_3D('',#10160,#7024,#7025);
#5678=AXIS2_PLACEMENT_3D('',#10161,#7026,#7027);
#5679=AXIS2_PLACEMENT_3D('',#10162,#7028,#7029);
#5680=AXIS2_PLACEMENT_3D('',#10186,#7030,#7031);
#5681=AXIS2_PLACEMENT_3D('',#10187,#7032,#7033);
#5682=AXIS2_PLACEMENT_3D('',#10189,#7034,#7035);
#5683=AXIS2_PLACEMENT_3D('',#10192,#7037,#7038);
#5684=AXIS2_PLACEMENT_3D('',#10216,#7039,#7040);
#5685=AXIS2_PLACEMENT_3D('',#10217,#7041,#7042);
#5686=AXIS2_PLACEMENT_3D('',#10218,#7043,#7044);
#5687=AXIS2_PLACEMENT_3D('',#10219,#7045,#7046);
#5688=AXIS2_PLACEMENT_3D('',#10220,#7047,#7048);
#5689=AXIS2_PLACEMENT_3D('',#10221,#7049,#7050);
#5690=AXIS2_PLACEMENT_3D('',#10222,#7051,#7052);
#6943=DIRECTION('axis',(0.,0.,1.));
#6944=DIRECTION('refdir',(1.,0.,0.));
#6945=DIRECTION('center_axis',(0.,0.,1.));
#6946=DIRECTION('ref_axis',(1.,0.,0.));
#6947=DIRECTION('center_axis',(0.,-1.,0.));
#6948=DIRECTION('ref_axis',(0.,0.,-1.));
#6949=DIRECTION('center_axis',(0.,-1.,0.));
#6950=DIRECTION('ref_axis',(0.,0.,-1.));
#6951=DIRECTION('center_axis',(0.,1.,0.));
#6952=DIRECTION('ref_axis',(1.,0.,0.));
#6953=DIRECTION('center_axis',(0.,1.,0.));
#6954=DIRECTION('ref_axis',(1.,0.,0.));
#6955=DIRECTION('center_axis',(0.,1.,0.));
#6956=DIRECTION('ref_axis',(1.,0.,0.));
#6957=DIRECTION('center_axis',(0.,1.,0.));
#6958=DIRECTION('ref_axis',(1.,0.,0.));
#6959=DIRECTION('',(0.,-1.,0.));
#6960=DIRECTION('center_axis',(0.,-1.,0.));
#6961=DIRECTION('ref_axis',(1.,0.,0.));
#6962=DIRECTION('center_axis',(0.,1.,0.));
#6963=DIRECTION('ref_axis',(1.,0.,0.));
#6964=DIRECTION('center_axis',(0.,1.,0.));
#6965=DIRECTION('ref_axis',(1.,0.,0.));
#6966=DIRECTION('center_axis',(0.,1.,0.));
#6967=DIRECTION('ref_axis',(1.,0.,0.));
#6968=DIRECTION('center_axis',(0.,1.,0.));
#6969=DIRECTION('ref_axis',(1.,0.,0.));
#6970=DIRECTION('center_axis',(0.,1.,0.));
#6971=DIRECTION('ref_axis',(1.,0.,0.));
#6972=DIRECTION('center_axis',(0.,1.,0.));
#6973=DIRECTION('ref_axis',(1.,0.,0.));
#6974=DIRECTION('center_axis',(0.,-1.,0.));
#6975=DIRECTION('ref_axis',(1.,0.,0.));
#6976=DIRECTION('center_axis',(0.,-1.,0.));
#6977=DIRECTION('ref_axis',(0.,0.,-1.));
#6978=DIRECTION('center_axis',(6.12323399573677E-17,0.,1.));
#6979=DIRECTION('ref_axis',(1.,0.,0.));
#6980=DIRECTION('center_axis',(0.,-1.,0.));
#6981=DIRECTION('ref_axis',(0.,0.,-1.));
#6982=DIRECTION('center_axis',(0.,1.,0.));
#6983=DIRECTION('ref_axis',(1.,0.,0.));
#6984=DIRECTION('center_axis',(0.,-1.,0.));
#6985=DIRECTION('ref_axis',(1.,0.,0.));
#6986=DIRECTION('center_axis',(0.,-1.,0.));
#6987=DIRECTION('ref_axis',(0.,0.,-1.));
#6988=DIRECTION('center_axis',(0.,0.,1.));
#6989=DIRECTION('ref_axis',(1.,0.,0.));
#6990=DIRECTION('center_axis',(0.,-1.,0.));
#6991=DIRECTION('ref_axis',(0.,0.,-1.));
#6992=DIRECTION('center_axis',(0.,1.,0.));
#6993=DIRECTION('ref_axis',(1.,0.,0.));
#6994=DIRECTION('center_axis',(0.,-1.,0.));
#6995=DIRECTION('ref_axis',(1.,0.,0.));
#6996=DIRECTION('center_axis',(0.,-1.,0.));
#6997=DIRECTION('ref_axis',(0.,0.,-1.));
#6998=DIRECTION('center_axis',(0.,0.,1.));
#6999=DIRECTION('ref_axis',(1.,0.,0.));
#7000=DIRECTION('center_axis',(0.,-1.,0.));
#7001=DIRECTION('ref_axis',(0.,0.,-1.));
#7002=DIRECTION('center_axis',(0.,1.,0.));
#7003=DIRECTION('ref_axis',(1.,0.,0.));
#7004=DIRECTION('center_axis',(0.,-1.,0.));
#7005=DIRECTION('ref_axis',(1.,0.,0.));
#7006=DIRECTION('center_axis',(0.,-1.,0.));
#7007=DIRECTION('ref_axis',(0.,0.,-1.));
#7008=DIRECTION('center_axis',(0.,0.,1.));
#7009=DIRECTION('ref_axis',(1.,0.,0.));
#7010=DIRECTION('center_axis',(0.,-1.,0.));
#7011=DIRECTION('ref_axis',(0.,0.,-1.));
#7012=DIRECTION('center_axis',(0.,1.,0.));
#7013=DIRECTION('ref_axis',(1.,0.,0.));
#7014=DIRECTION('center_axis',(0.,-1.,0.));
#7015=DIRECTION('ref_axis',(1.,0.,0.));
#7016=DIRECTION('center_axis',(0.,-1.,0.));
#7017=DIRECTION('ref_axis',(0.,0.,-1.));
#7018=DIRECTION('center_axis',(6.12323399573676E-17,0.,1.));
#7019=DIRECTION('ref_axis',(1.,0.,0.));
#7020=DIRECTION('center_axis',(0.,-1.,0.));
#7021=DIRECTION('ref_axis',(0.,0.,-1.));
#7022=DIRECTION('center_axis',(0.,1.,0.));
#7023=DIRECTION('ref_axis',(1.,0.,0.));
#7024=DIRECTION('center_axis',(0.,-1.,0.));
#7025=DIRECTION('ref_axis',(1.,0.,0.));
#7026=DIRECTION('center_axis',(0.,-1.,0.));
#7027=DIRECTION('ref_axis',(0.,0.,-1.));
#7028=DIRECTION('center_axis',(0.,0.,1.));
#7029=DIRECTION('ref_axis',(1.,0.,0.));
#7030=DIRECTION('center_axis',(0.,-1.,0.));
#7031=DIRECTION('ref_axis',(0.,0.,-1.));
#7032=DIRECTION('center_axis',(0.,1.,0.));
#7033=DIRECTION('ref_axis',(1.,0.,0.));
#7034=DIRECTION('center_axis',(0.,1.,0.));
#7035=DIRECTION('ref_axis',(1.,0.,0.));
#7036=DIRECTION('',(0.,1.,0.));
#7037=DIRECTION('center_axis',(0.,-1.,0.));
#7038=DIRECTION('ref_axis',(1.,0.,0.));
#7039=DIRECTION('center_axis',(0.,-1.,0.));
#7040=DIRECTION('ref_axis',(1.,0.,0.));
#7041=DIRECTION('center_axis',(0.,1.,0.));
#7042=DIRECTION('ref_axis',(1.,0.,0.));
#7043=DIRECTION('center_axis',(0.,-1.,0.));
#7044=DIRECTION('ref_axis',(0.,0.,-1.));
#7045=DIRECTION('center_axis',(0.,0.,1.));
#7046=DIRECTION('ref_axis',(1.,0.,0.));
#7047=DIRECTION('center_axis',(0.,-1.,0.));
#7048=DIRECTION('ref_axis',(0.,0.,-1.));
#7049=DIRECTION('center_axis',(0.,-1.,0.));
#7050=DIRECTION('ref_axis',(-1.,0.,0.));
#7051=DIRECTION('center_axis',(0.,1.,0.));
#7052=DIRECTION('ref_axis',(1.,0.,0.));
#9775=CARTESIAN_POINT('',(0.,0.,0.));
#9776=CARTESIAN_POINT('Origin',(0.707106781186547,0.,0.707106781186548));
#9777=CARTESIAN_POINT('',(0.504455939115715,-0.04763,0.841298510752802));
#9778=CARTESIAN_POINT('',(0.841298510752802,-0.04763,0.504455939115715));
#9779=CARTESIAN_POINT('Ctrl Pts',(0.504455939115715,-0.04763,0.841298510752802));
#9780=CARTESIAN_POINT('Ctrl Pts',(0.508899795931835,-0.0740444353928835,
0.838633903678357));
#9781=CARTESIAN_POINT('Ctrl Pts',(0.517157748491652,-0.0999305678883309,
0.833661031856294));
#9782=CARTESIAN_POINT('Ctrl Pts',(0.537715343527944,-0.142345102874864,
0.820511285096538));
#9783=CARTESIAN_POINT('Ctrl Pts',(0.548874290046456,-0.159766064500479,
0.813159949759));
#9784=CARTESIAN_POINT('Ctrl Pts',(0.573915184558107,-0.190326085855194,
0.795684265985089));
#9785=CARTESIAN_POINT('Ctrl Pts',(0.587792702767295,-0.203463743702801,
0.78555112003688));
#9786=CARTESIAN_POINT('Ctrl Pts',(0.615966552324775,-0.224161999508995,
0.763642258217233));
#9787=CARTESIAN_POINT('Ctrl Pts',(0.631684198665438,-0.232861760990032,
0.750785745543687));
#9788=CARTESIAN_POINT('Ctrl Pts',(0.663382628119203,-0.244251601209411,
0.722929908501543));
#9789=CARTESIAN_POINT('Ctrl Pts',(0.679352081686668,-0.246942143572133,
0.707917883896095));
#9790=CARTESIAN_POINT('Ctrl Pts',(0.707917883896095,-0.246942143572133,
0.679352081686668));
#9791=CARTESIAN_POINT('Ctrl Pts',(0.722929908501543,-0.244251601209411,
0.663382628119203));
#9792=CARTESIAN_POINT('Ctrl Pts',(0.750785745543687,-0.232861760990032,
0.631684198665439));
#9793=CARTESIAN_POINT('Ctrl Pts',(0.763642258217232,-0.224161999508995,
0.615966552324775));
#9794=CARTESIAN_POINT('Ctrl Pts',(0.78555112003688,-0.203463743702801,0.587792702767295));
#9795=CARTESIAN_POINT('Ctrl Pts',(0.795684265985088,-0.190326085855194,
0.573915184558108));
#9796=CARTESIAN_POINT('Ctrl Pts',(0.813159949759,-0.15976606450048,0.548874290046456));
#9797=CARTESIAN_POINT('Ctrl Pts',(0.820511285096538,-0.142345102874864,
0.537715343527944));
#9798=CARTESIAN_POINT('Ctrl Pts',(0.833661031856294,-0.099930567888331,
0.517157748491653));
#9799=CARTESIAN_POINT('Ctrl Pts',(0.838633903678357,-0.0740444353928835,
0.508899795931835));
#9800=CARTESIAN_POINT('Ctrl Pts',(0.841298510752801,-0.0476299999999999,
0.504455939115715));
#9801=CARTESIAN_POINT('',(0.528110872004958,-0.04763,0.871530771444223));
#9802=CARTESIAN_POINT('Origin',(0.707106781186547,-0.04763,0.707106781186548));
#9803=CARTESIAN_POINT('',(0.871530771444223,-0.04763,0.528110872004959));
#9804=CARTESIAN_POINT('Ctrl Pts',(0.871530771444223,-0.0476300000000001,
0.528110872004958));
#9805=CARTESIAN_POINT('Ctrl Pts',(0.87014664509073,-0.0609922781173483,
0.530395067942936));
#9806=CARTESIAN_POINT('Ctrl Pts',(0.868149331745851,-0.0742967091364493,
0.533674141594226));
#9807=CARTESIAN_POINT('Ctrl Pts',(0.85981294420286,-0.115492077056649,0.54708917182331));
#9808=CARTESIAN_POINT('Ctrl Pts',(0.850993704737257,-0.141695629206859,
0.560922177770136));
#9809=CARTESIAN_POINT('Ctrl Pts',(0.830754510485543,-0.181890537957859,
0.590422647829571));
#9810=CARTESIAN_POINT('Ctrl Pts',(0.816896541396381,-0.201072148666545,
0.609616703125488));
#9811=CARTESIAN_POINT('Ctrl Pts',(0.792310597819928,-0.223955109275652,
0.641117951819998));
#9812=CARTESIAN_POINT('Ctrl Pts',(0.779109323683612,-0.232742381310829,
0.657208095763053));
#9813=CARTESIAN_POINT('Ctrl Pts',(0.750552691816206,-0.244234834628584,
0.68964083160521));
#9814=CARTESIAN_POINT('Ctrl Pts',(0.735185187071673,-0.246942143572133,
0.705971972091755));
#9815=CARTESIAN_POINT('Ctrl Pts',(0.705971972091754,-0.246942143572133,
0.735185187071673));
#9816=CARTESIAN_POINT('Ctrl Pts',(0.689640831605209,-0.244234834628584,
0.750552691816206));
#9817=CARTESIAN_POINT('Ctrl Pts',(0.657208095763052,-0.232742381310829,
0.779109323683612));
#9818=CARTESIAN_POINT('Ctrl Pts',(0.641117951819998,-0.223955109275652,
0.792310597819928));
#9819=CARTESIAN_POINT('Ctrl Pts',(0.609616703125487,-0.201072148666545,
0.816896541396382));
#9820=CARTESIAN_POINT('Ctrl Pts',(0.590422647829571,-0.181890537957858,
0.830754510485544));
#9821=CARTESIAN_POINT('Ctrl Pts',(0.560922177770135,-0.141695629206858,
0.850993704737257));
#9822=CARTESIAN_POINT('Ctrl Pts',(0.547089171823309,-0.115492077056649,
0.859812944202861));
#9823=CARTESIAN_POINT('Ctrl Pts',(0.533674141594226,-0.0742967091364491,
0.868149331745852));
#9824=CARTESIAN_POINT('Ctrl Pts',(0.530395067942936,-0.0609922781173483,
0.870146645090731));
#9825=CARTESIAN_POINT('Ctrl Pts',(0.528110872004958,-0.0476300000000001,
0.871530771444223));
#9826=CARTESIAN_POINT('Origin',(0.707106781186547,-0.04763,0.707106781186548));
#9827=CARTESIAN_POINT('Origin',(0.,-0.166705,0.));
#9828=CARTESIAN_POINT('',(0.242834539687906,-0.04763,0.989696097314));
#9829=CARTESIAN_POINT('Origin',(0.,-0.04763,0.));
#9830=CARTESIAN_POINT('',(-0.242834539687907,-0.04763,0.989696097314));
#9831=CARTESIAN_POINT('Ctrl Pts',(0.242834539687906,-0.04763,0.989696097314));
#9832=CARTESIAN_POINT('Ctrl Pts',(0.24024064412003,-0.0609922781173483,
0.990332542620729));
#9833=CARTESIAN_POINT('Ctrl Pts',(0.236509675094874,-0.0742967091364492,
0.991238884025248));
#9834=CARTESIAN_POINT('Ctrl Pts',(0.221129100087819,-0.115492077056649,
0.994830026707808));
#9835=CARTESIAN_POINT('Ctrl Pts',(0.205111543747588,-0.141695629206859,
0.998375294985966));
#9836=CARTESIAN_POINT('Ctrl Pts',(0.169940289819232,-0.181890537957859,
1.00492400591205));
#9837=CARTESIAN_POINT('Ctrl Pts',(0.1465689792446,-0.201072148666545,1.00869718865384));
#9838=CARTESIAN_POINT('Ctrl Pts',(0.106909345252087,-0.223955109275652,
1.01358704779679));
#9839=CARTESIAN_POINT('Ctrl Pts',(0.0861971848975941,-0.232742381310829,
1.0156297872271));
#9840=CARTESIAN_POINT('Ctrl Pts',(0.0430711894098822,-0.244234834628584,
1.01837060663223));
#9841=CARTESIAN_POINT('Ctrl Pts',(0.0206568624125605,-0.246942143572133,
1.019052));
#9842=CARTESIAN_POINT('Ctrl Pts',(-0.0206568624125608,-0.246942143572133,
1.019052));
#9843=CARTESIAN_POINT('Ctrl Pts',(-0.0430711894098825,-0.244234834628584,
1.01837060663223));
#9844=CARTESIAN_POINT('Ctrl Pts',(-0.0861971848975943,-0.232742381310829,
1.0156297872271));
#9845=CARTESIAN_POINT('Ctrl Pts',(-0.106909345252088,-0.223955109275652,
1.01358704779679));
#9846=CARTESIAN_POINT('Ctrl Pts',(-0.1465689792446,-0.201072148666545,1.00869718865384));
#9847=CARTESIAN_POINT('Ctrl Pts',(-0.169940289819232,-0.181890537957859,
1.00492400591205));
#9848=CARTESIAN_POINT('Ctrl Pts',(-0.205111543747588,-0.141695629206859,
0.998375294985966));
#9849=CARTESIAN_POINT('Ctrl Pts',(-0.221129100087819,-0.115492077056649,
0.994830026707808));
#9850=CARTESIAN_POINT('Ctrl Pts',(-0.236509675094875,-0.0742967091364493,
0.991238884025248));
#9851=CARTESIAN_POINT('Ctrl Pts',(-0.24024064412003,-0.0609922781173483,
0.990332542620729));
#9852=CARTESIAN_POINT('Ctrl Pts',(-0.242834539687907,-0.04763,0.989696097314));
#9853=CARTESIAN_POINT('',(-0.528110872004959,-0.04763,0.871530771444223));
#9854=CARTESIAN_POINT('Origin',(0.,-0.04763,0.));
#9855=CARTESIAN_POINT('',(-0.871530771444223,-0.04763,0.528110872004958));
#9856=CARTESIAN_POINT('Ctrl Pts',(-0.528110872004958,-0.0476300000000001,
0.871530771444223));
#9857=CARTESIAN_POINT('Ctrl Pts',(-0.530395067942936,-0.0609922781173484,
0.87014664509073));
#9858=CARTESIAN_POINT('Ctrl Pts',(-0.533674141594226,-0.0742967091364493,
0.868149331745851));
#9859=CARTESIAN_POINT('Ctrl Pts',(-0.54708917182331,-0.115492077056649,
0.85981294420286));
#9860=CARTESIAN_POINT('Ctrl Pts',(-0.560922177770136,-0.141695629206859,
0.850993704737257));
#9861=CARTESIAN_POINT('Ctrl Pts',(-0.590422647829571,-0.181890537957859,
0.830754510485543));
#9862=CARTESIAN_POINT('Ctrl Pts',(-0.609616703125488,-0.201072148666545,
0.816896541396381));
#9863=CARTESIAN_POINT('Ctrl Pts',(-0.641117951819998,-0.223955109275652,
0.792310597819928));
#9864=CARTESIAN_POINT('Ctrl Pts',(-0.657208095763053,-0.232742381310829,
0.779109323683611));
#9865=CARTESIAN_POINT('Ctrl Pts',(-0.68964083160521,-0.244234834628584,
0.750552691816205));
#9866=CARTESIAN_POINT('Ctrl Pts',(-0.705971972091755,-0.246942143572133,
0.735185187071673));
#9867=CARTESIAN_POINT('Ctrl Pts',(-0.735185187071673,-0.246942143572133,
0.705971972091754));
#9868=CARTESIAN_POINT('Ctrl Pts',(-0.750552691816206,-0.244234834628584,
0.689640831605209));
#9869=CARTESIAN_POINT('Ctrl Pts',(-0.779109323683612,-0.232742381310829,
0.657208095763052));
#9870=CARTESIAN_POINT('Ctrl Pts',(-0.792310597819928,-0.223955109275652,
0.641117951819998));
#9871=CARTESIAN_POINT('Ctrl Pts',(-0.816896541396382,-0.201072148666545,
0.609616703125487));
#9872=CARTESIAN_POINT('Ctrl Pts',(-0.830754510485544,-0.181890537957858,
0.590422647829571));
#9873=CARTESIAN_POINT('Ctrl Pts',(-0.850993704737257,-0.141695629206858,
0.560922177770135));
#9874=CARTESIAN_POINT('Ctrl Pts',(-0.859812944202861,-0.115492077056649,
0.547089171823309));
#9875=CARTESIAN_POINT('Ctrl Pts',(-0.868149331745852,-0.0742967091364491,
0.533674141594226));
#9876=CARTESIAN_POINT('Ctrl Pts',(-0.870146645090731,-0.0609922781173483,
0.530395067942936));
#9877=CARTESIAN_POINT('Ctrl Pts',(-0.871530771444223,-0.04763,0.528110872004958));
#9878=CARTESIAN_POINT('',(-0.989696097314,-0.04763,0.242834539687906));
#9879=CARTESIAN_POINT('Origin',(0.,-0.04763,0.));
#9880=CARTESIAN_POINT('',(-1.019052,-0.246942143572133,1.248489836334E-16));
#9881=CARTESIAN_POINT('Ctrl Pts',(-0.989696097314,-0.04763,0.242834539687906));
#9882=CARTESIAN_POINT('Ctrl Pts',(-0.990332542620729,-0.0609922781173483,
0.24024064412003));
#9883=CARTESIAN_POINT('Ctrl Pts',(-0.991238884025248,-0.0742967091364492,
0.236509675094874));
#9884=CARTESIAN_POINT('Ctrl Pts',(-0.994830026707808,-0.115492077056649,
0.221129100087819));
#9885=CARTESIAN_POINT('Ctrl Pts',(-0.998375294985966,-0.141695629206859,
0.205111543747588));
#9886=CARTESIAN_POINT('Ctrl Pts',(-1.00492400591205,-0.181890537957859,
0.169940289819232));
#9887=CARTESIAN_POINT('Ctrl Pts',(-1.00869718865384,-0.201072148666545,
0.1465689792446));
#9888=CARTESIAN_POINT('Ctrl Pts',(-1.01358704779679,-0.223955109275652,
0.106909345252088));
#9889=CARTESIAN_POINT('Ctrl Pts',(-1.0156297872271,-0.232742381310829,0.0861971848975944));
#9890=CARTESIAN_POINT('Ctrl Pts',(-1.01837060663223,-0.244234834628584,
0.0430711894098825));
#9891=CARTESIAN_POINT('Ctrl Pts',(-1.019052,-0.246942143572133,0.0206568624125608));
#9892=CARTESIAN_POINT('Ctrl Pts',(-1.019052,-0.246942143572133,1.2490009027033E-16));
#9893=CARTESIAN_POINT('',(-1.019052,-0.28578,1.24797876996471E-16));
#9894=CARTESIAN_POINT('',(-1.019052,-0.166705,1.24797876996471E-16));
#9895=CARTESIAN_POINT('Origin',(0.,-0.28578,0.));
#9896=CARTESIAN_POINT('',(-0.989696097314,-0.04763,-0.242834539687906));
#9897=CARTESIAN_POINT('Ctrl Pts',(-1.019052,-0.246942143572133,1.2490009027033E-16));
#9898=CARTESIAN_POINT('Ctrl Pts',(-1.019052,-0.246942143572133,-0.0206568624125605));
#9899=CARTESIAN_POINT('Ctrl Pts',(-1.01837060663223,-0.244234834628584,
-0.0430711894098822));
#9900=CARTESIAN_POINT('Ctrl Pts',(-1.0156297872271,-0.232742381310829,-0.0861971848975941));
#9901=CARTESIAN_POINT('Ctrl Pts',(-1.01358704779679,-0.223955109275652,
-0.106909345252087));
#9902=CARTESIAN_POINT('Ctrl Pts',(-1.00869718865384,-0.201072148666546,
-0.1465689792446));
#9903=CARTESIAN_POINT('Ctrl Pts',(-1.00492400591205,-0.181890537957859,
-0.169940289819232));
#9904=CARTESIAN_POINT('Ctrl Pts',(-0.998375294985966,-0.141695629206859,
-0.205111543747588));
#9905=CARTESIAN_POINT('Ctrl Pts',(-0.994830026707808,-0.11549207705665,
-0.221129100087819));
#9906=CARTESIAN_POINT('Ctrl Pts',(-0.991238884025248,-0.0742967091364495,
-0.236509675094874));
#9907=CARTESIAN_POINT('Ctrl Pts',(-0.990332542620729,-0.0609922781173484,
-0.24024064412003));
#9908=CARTESIAN_POINT('Ctrl Pts',(-0.989696097314,-0.0476300000000001,-0.242834539687907));
#9909=CARTESIAN_POINT('',(-0.871530771444223,-0.04763,-0.528110872004958));
#9910=CARTESIAN_POINT('Origin',(0.,-0.04763,0.));
#9911=CARTESIAN_POINT('',(-0.528110872004958,-0.04763,-0.871530771444223));
#9912=CARTESIAN_POINT('Ctrl Pts',(-0.871530771444223,-0.0476300000000001,
-0.528110872004958));
#9913=CARTESIAN_POINT('Ctrl Pts',(-0.87014664509073,-0.0609922781173484,
-0.530395067942936));
#9914=CARTESIAN_POINT('Ctrl Pts',(-0.868149331745851,-0.0742967091364494,
-0.533674141594226));
#9915=CARTESIAN_POINT('Ctrl Pts',(-0.85981294420286,-0.115492077056649,
-0.54708917182331));
#9916=CARTESIAN_POINT('Ctrl Pts',(-0.850993704737257,-0.141695629206859,
-0.560922177770136));
#9917=CARTESIAN_POINT('Ctrl Pts',(-0.830754510485543,-0.181890537957859,
-0.590422647829571));
#9918=CARTESIAN_POINT('Ctrl Pts',(-0.816896541396381,-0.201072148666546,
-0.609616703125488));
#9919=CARTESIAN_POINT('Ctrl Pts',(-0.792310597819928,-0.223955109275652,
-0.641117951819999));
#9920=CARTESIAN_POINT('Ctrl Pts',(-0.779109323683611,-0.232742381310829,
-0.657208095763053));
#9921=CARTESIAN_POINT('Ctrl Pts',(-0.750552691816205,-0.244234834628584,
-0.68964083160521));
#9922=CARTESIAN_POINT('Ctrl Pts',(-0.735185187071673,-0.246942143572133,
-0.705971972091755));
#9923=CARTESIAN_POINT('Ctrl Pts',(-0.705971972091754,-0.246942143572133,
-0.735185187071673));
#9924=CARTESIAN_POINT('Ctrl Pts',(-0.68964083160521,-0.244234834628584,
-0.750552691816206));
#9925=CARTESIAN_POINT('Ctrl Pts',(-0.657208095763052,-0.232742381310829,
-0.779109323683612));
#9926=CARTESIAN_POINT('Ctrl Pts',(-0.641117951819998,-0.223955109275652,
-0.792310597819928));
#9927=CARTESIAN_POINT('Ctrl Pts',(-0.609616703125488,-0.201072148666545,
-0.816896541396381));
#9928=CARTESIAN_POINT('Ctrl Pts',(-0.590422647829571,-0.181890537957859,
-0.830754510485543));
#9929=CARTESIAN_POINT('Ctrl Pts',(-0.560922177770136,-0.141695629206859,
-0.850993704737257));
#9930=CARTESIAN_POINT('Ctrl Pts',(-0.54708917182331,-0.115492077056649,
-0.85981294420286));
#9931=CARTESIAN_POINT('Ctrl Pts',(-0.533674141594226,-0.0742967091364494,
-0.868149331745852));
#9932=CARTESIAN_POINT('Ctrl Pts',(-0.530395067942936,-0.0609922781173484,
-0.870146645090731));
#9933=CARTESIAN_POINT('Ctrl Pts',(-0.528110872004958,-0.0476300000000001,
-0.871530771444223));
#9934=CARTESIAN_POINT('',(-0.242834539687906,-0.04763,-0.989696097314));
#9935=CARTESIAN_POINT('Origin',(0.,-0.04763,0.));
#9936=CARTESIAN_POINT('',(0.242834539687906,-0.04763,-0.989696097314));
#9937=CARTESIAN_POINT('Ctrl Pts',(-0.242834539687907,-0.04763,-0.989696097314));
#9938=CARTESIAN_POINT('Ctrl Pts',(-0.24024064412003,-0.0609922781173483,
-0.990332542620729));
#9939=CARTESIAN_POINT('Ctrl Pts',(-0.236509675094874,-0.0742967091364493,
-0.991238884025248));
#9940=CARTESIAN_POINT('Ctrl Pts',(-0.221129100087819,-0.115492077056649,
-0.994830026707808));
#9941=CARTESIAN_POINT('Ctrl Pts',(-0.205111543747588,-0.141695629206859,
-0.998375294985966));
#9942=CARTESIAN_POINT('Ctrl Pts',(-0.169940289819232,-0.181890537957859,
-1.00492400591205));
#9943=CARTESIAN_POINT('Ctrl Pts',(-0.1465689792446,-0.201072148666545,-1.00869718865384));
#9944=CARTESIAN_POINT('Ctrl Pts',(-0.106909345252087,-0.223955109275652,
-1.01358704779679));
#9945=CARTESIAN_POINT('Ctrl Pts',(-0.0861971848975942,-0.232742381310829,
-1.0156297872271));
#9946=CARTESIAN_POINT('Ctrl Pts',(-0.0430711894098823,-0.244234834628584,
-1.01837060663223));
#9947=CARTESIAN_POINT('Ctrl Pts',(-0.0206568624125606,-0.246942143572133,
-1.019052));
#9948=CARTESIAN_POINT('Ctrl Pts',(0.0206568624125607,-0.246942143572133,
-1.019052));
#9949=CARTESIAN_POINT('Ctrl Pts',(0.0430711894098824,-0.244234834628584,
-1.01837060663223));
#9950=CARTESIAN_POINT('Ctrl Pts',(0.0861971848975943,-0.232742381310829,
-1.0156297872271));
#9951=CARTESIAN_POINT('Ctrl Pts',(0.106909345252088,-0.223955109275652,
-1.01358704779679));
#9952=CARTESIAN_POINT('Ctrl Pts',(0.1465689792446,-0.201072148666545,-1.00869718865384));
#9953=CARTESIAN_POINT('Ctrl Pts',(0.169940289819232,-0.181890537957859,
-1.00492400591205));
#9954=CARTESIAN_POINT('Ctrl Pts',(0.205111543747588,-0.141695629206859,
-0.998375294985966));
#9955=CARTESIAN_POINT('Ctrl Pts',(0.221129100087819,-0.115492077056649,
-0.994830026707808));
#9956=CARTESIAN_POINT('Ctrl Pts',(0.236509675094874,-0.0742967091364493,
-0.991238884025248));
#9957=CARTESIAN_POINT('Ctrl Pts',(0.24024064412003,-0.0609922781173484,
-0.990332542620729));
#9958=CARTESIAN_POINT('Ctrl Pts',(0.242834539687907,-0.04763,-0.989696097314));
#9959=CARTESIAN_POINT('',(0.528110872004958,-0.04763,-0.871530771444223));
#9960=CARTESIAN_POINT('Origin',(0.,-0.04763,0.));
#9961=CARTESIAN_POINT('',(0.871530771444223,-0.04763,-0.528110872004958));
#9962=CARTESIAN_POINT('Ctrl Pts',(0.528110872004958,-0.0476300000000001,
-0.871530771444223));
#9963=CARTESIAN_POINT('Ctrl Pts',(0.530395067942936,-0.0609922781173484,
-0.870146645090731));
#9964=CARTESIAN_POINT('Ctrl Pts',(0.533674141594226,-0.0742967091364493,
-0.868149331745851));
#9965=CARTESIAN_POINT('Ctrl Pts',(0.54708917182331,-0.115492077056649,-0.85981294420286));
#9966=CARTESIAN_POINT('Ctrl Pts',(0.560922177770136,-0.141695629206859,
-0.850993704737257));
#9967=CARTESIAN_POINT('Ctrl Pts',(0.590422647829571,-0.181890537957859,
-0.830754510485543));
#9968=CARTESIAN_POINT('Ctrl Pts',(0.609616703125488,-0.201072148666545,
-0.816896541396381));
#9969=CARTESIAN_POINT('Ctrl Pts',(0.641117951819998,-0.223955109275652,
-0.792310597819928));
#9970=CARTESIAN_POINT('Ctrl Pts',(0.657208095763053,-0.232742381310829,
-0.779109323683612));
#9971=CARTESIAN_POINT('Ctrl Pts',(0.68964083160521,-0.244234834628584,-0.750552691816206));
#9972=CARTESIAN_POINT('Ctrl Pts',(0.705971972091755,-0.246942143572133,
-0.735185187071673));
#9973=CARTESIAN_POINT('Ctrl Pts',(0.735185187071673,-0.246942143572133,
-0.705971972091754));
#9974=CARTESIAN_POINT('Ctrl Pts',(0.750552691816206,-0.244234834628584,
-0.68964083160521));
#9975=CARTESIAN_POINT('Ctrl Pts',(0.779109323683612,-0.232742381310829,
-0.657208095763053));
#9976=CARTESIAN_POINT('Ctrl Pts',(0.792310597819928,-0.223955109275652,
-0.641117951819998));
#9977=CARTESIAN_POINT('Ctrl Pts',(0.816896541396381,-0.201072148666545,
-0.609616703125488));
#9978=CARTESIAN_POINT('Ctrl Pts',(0.830754510485543,-0.181890537957859,
-0.590422647829571));
#9979=CARTESIAN_POINT('Ctrl Pts',(0.850993704737257,-0.141695629206859,
-0.560922177770136));
#9980=CARTESIAN_POINT('Ctrl Pts',(0.85981294420286,-0.115492077056649,-0.54708917182331));
#9981=CARTESIAN_POINT('Ctrl Pts',(0.868149331745851,-0.0742967091364493,
-0.533674141594226));
#9982=CARTESIAN_POINT('Ctrl Pts',(0.870146645090731,-0.0609922781173484,
-0.530395067942936));
#9983=CARTESIAN_POINT('Ctrl Pts',(0.871530771444223,-0.0476300000000001,
-0.528110872004958));
#9984=CARTESIAN_POINT('',(0.989696097314,-0.04763,-0.242834539687906));
#9985=CARTESIAN_POINT('Origin',(0.,-0.04763,0.));
#9986=CARTESIAN_POINT('',(0.989696097314,-0.04763,0.242834539687906));
#9987=CARTESIAN_POINT('Ctrl Pts',(0.989696097314,-0.04763,-0.242834539687907));
#9988=CARTESIAN_POINT('Ctrl Pts',(0.990332542620729,-0.0609922781173483,
-0.24024064412003));
#9989=CARTESIAN_POINT('Ctrl Pts',(0.991238884025248,-0.0742967091364493,
-0.236509675094874));
#9990=CARTESIAN_POINT('Ctrl Pts',(0.994830026707808,-0.115492077056649,
-0.221129100087819));
#9991=CARTESIAN_POINT('Ctrl Pts',(0.998375294985966,-0.141695629206859,
-0.205111543747588));
#9992=CARTESIAN_POINT('Ctrl Pts',(1.00492400591205,-0.181890537957859,-0.169940289819232));
#9993=CARTESIAN_POINT('Ctrl Pts',(1.00869718865384,-0.201072148666545,-0.1465689792446));
#9994=CARTESIAN_POINT('Ctrl Pts',(1.01358704779679,-0.223955109275652,-0.106909345252087));
#9995=CARTESIAN_POINT('Ctrl Pts',(1.0156297872271,-0.232742381310829,-0.0861971848975942));
#9996=CARTESIAN_POINT('Ctrl Pts',(1.01837060663223,-0.244234834628584,-0.0430711894098823));
#9997=CARTESIAN_POINT('Ctrl Pts',(1.019052,-0.246942143572133,-0.0206568624125607));
#9998=CARTESIAN_POINT('Ctrl Pts',(1.019052,-0.246942143572133,0.0206568624125607));
#9999=CARTESIAN_POINT('Ctrl Pts',(1.01837060663223,-0.244234834628584,0.0430711894098823));
#10000=CARTESIAN_POINT('Ctrl Pts',(1.0156297872271,-0.232742381310829,0.0861971848975942));
#10001=CARTESIAN_POINT('Ctrl Pts',(1.01358704779679,-0.223955109275652,
0.106909345252087));
#10002=CARTESIAN_POINT('Ctrl Pts',(1.00869718865384,-0.201072148666545,
0.1465689792446));
#10003=CARTESIAN_POINT('Ctrl Pts',(1.00492400591205,-0.181890537957859,
0.169940289819232));
#10004=CARTESIAN_POINT('Ctrl Pts',(0.998375294985966,-0.141695629206859,
0.205111543747588));
#10005=CARTESIAN_POINT('Ctrl Pts',(0.994830026707808,-0.115492077056649,
0.221129100087819));
#10006=CARTESIAN_POINT('Ctrl Pts',(0.991238884025248,-0.0742967091364492,
0.236509675094874));
#10007=CARTESIAN_POINT('Ctrl Pts',(0.990332542620729,-0.0609922781173483,
0.24024064412003));
#10008=CARTESIAN_POINT('Ctrl Pts',(0.989696097314,-0.04763,0.242834539687907));
#10009=CARTESIAN_POINT('Origin',(0.,-0.04763,0.));
#10010=CARTESIAN_POINT('Origin',(0.,-0.04763,0.));
#10011=CARTESIAN_POINT('',(0.238183666596899,-0.04763,0.951592097314));
#10012=CARTESIAN_POINT('Origin',(0.,-0.04763,0.));
#10013=CARTESIAN_POINT('Origin',(-1.94289029309402E-16,-0.04763,1.));
#10014=CARTESIAN_POINT('Origin',(-1.94289029309402E-16,0.,1.));
#10015=CARTESIAN_POINT('',(-0.2381836665969,-0.04763,0.951592097314));
#10016=CARTESIAN_POINT('Ctrl Pts',(-0.238183666596899,-0.0476299999999999,
0.951592097314));
#10017=CARTESIAN_POINT('Ctrl Pts',(-0.233157223576062,-0.0740444353928835,
0.952850216871763));
#10018=CARTESIAN_POINT('Ctrl Pts',(-0.223801617934946,-0.0999305678883309,
0.955173119738174));
#10019=CARTESIAN_POINT('Ctrl Pts',(-0.199966927975188,-0.142345102874864,
0.960411259488514));
#10020=CARTESIAN_POINT('Ctrl Pts',(-0.1868781821531,-0.159766064500479,
0.963103647174702));
#10021=CARTESIAN_POINT('Ctrl Pts',(-0.15681442133453,-0.190326085855194,
0.968453058988463));
#10022=CARTESIAN_POINT('Ctrl Pts',(-0.139836317888043,-0.203463743702801,
0.971100730005489));
#10023=CARTESIAN_POINT('Ctrl Pts',(-0.104422493053067,-0.224161999508995,
0.975530745318961));
#10024=CARTESIAN_POINT('Ctrl Pts',(-0.0842175114474176,-0.232861760990032,
0.977553872336861));
#10025=CARTESIAN_POINT('Ctrl Pts',(-0.0421062857595701,-0.244251601209411,
0.980270995488453));
#10026=CARTESIAN_POINT('Ctrl Pts',(-0.0201990724523197,-0.246942143572133,
0.980948));
#10027=CARTESIAN_POINT('Ctrl Pts',(0.020199072452319,-0.246942143572133,
0.980948));
#10028=CARTESIAN_POINT('Ctrl Pts',(0.0421062857595694,-0.244251601209411,
0.980270995488454));
#10029=CARTESIAN_POINT('Ctrl Pts',(0.0842175114474169,-0.232861760990032,
0.977553872336861));
#10030=CARTESIAN_POINT('Ctrl Pts',(0.104422493053067,-0.224161999508995,
0.975530745318961));
#10031=CARTESIAN_POINT('Ctrl Pts',(0.139836317888042,-0.203463743702801,
0.971100730005489));
#10032=CARTESIAN_POINT('Ctrl Pts',(0.15681442133453,-0.190326085855194,
0.968453058988463));
#10033=CARTESIAN_POINT('Ctrl Pts',(0.1868781821531,-0.15976606450048,0.963103647174702));
#10034=CARTESIAN_POINT('Ctrl Pts',(0.199966927975188,-0.142345102874864,
0.960411259488514));
#10035=CARTESIAN_POINT('Ctrl Pts',(0.223801617934945,-0.0999305678883309,
0.955173119738174));
#10036=CARTESIAN_POINT('Ctrl Pts',(0.233157223576061,-0.0740444353928835,
0.952850216871763));
#10037=CARTESIAN_POINT('Ctrl Pts',(0.238183666596899,-0.0476299999999999,
0.951592097314));
#10038=CARTESIAN_POINT('Origin',(-1.94289029309402E-16,-0.04763,1.));
#10039=CARTESIAN_POINT('Origin',(0.,-0.04763,0.));
#10040=CARTESIAN_POINT('',(-0.504455939115715,-0.04763,0.841298510752802));
#10041=CARTESIAN_POINT('Origin',(0.,-0.04763,0.));
#10042=CARTESIAN_POINT('Origin',(-0.707106781186548,-0.04763,0.707106781186547));
#10043=CARTESIAN_POINT('Origin',(-0.707106781186548,0.,0.707106781186547));
#10044=CARTESIAN_POINT('',(-0.841298510752802,-0.04763,0.504455939115715));
#10045=CARTESIAN_POINT('Ctrl Pts',(-0.841298510752802,-0.04763,0.504455939115715));
#10046=CARTESIAN_POINT('Ctrl Pts',(-0.838633903678357,-0.0740444353928835,
0.508899795931835));
#10047=CARTESIAN_POINT('Ctrl Pts',(-0.833661031856294,-0.0999305678883309,
0.517157748491652));
#10048=CARTESIAN_POINT('Ctrl Pts',(-0.820511285096538,-0.142345102874864,
0.537715343527944));
#10049=CARTESIAN_POINT('Ctrl Pts',(-0.813159949759,-0.159766064500479,0.548874290046456));
#10050=CARTESIAN_POINT('Ctrl Pts',(-0.795684265985089,-0.190326085855194,
0.573915184558107));
#10051=CARTESIAN_POINT('Ctrl Pts',(-0.78555112003688,-0.203463743702801,
0.587792702767295));
#10052=CARTESIAN_POINT('Ctrl Pts',(-0.763642258217233,-0.224161999508995,
0.615966552324775));
#10053=CARTESIAN_POINT('Ctrl Pts',(-0.750785745543687,-0.232861760990032,
0.631684198665438));
#10054=CARTESIAN_POINT('Ctrl Pts',(-0.722929908501543,-0.244251601209411,
0.663382628119203));
#10055=CARTESIAN_POINT('Ctrl Pts',(-0.707917883896095,-0.246942143572133,
0.679352081686668));
#10056=CARTESIAN_POINT('Ctrl Pts',(-0.679352081686668,-0.246942143572133,
0.707917883896095));
#10057=CARTESIAN_POINT('Ctrl Pts',(-0.663382628119203,-0.244251601209411,
0.722929908501544));
#10058=CARTESIAN_POINT('Ctrl Pts',(-0.631684198665438,-0.232861760990031,
0.750785745543687));
#10059=CARTESIAN_POINT('Ctrl Pts',(-0.615966552324775,-0.224161999508995,
0.763642258217233));
#10060=CARTESIAN_POINT('Ctrl Pts',(-0.587792702767295,-0.203463743702801,
0.78555112003688));
#10061=CARTESIAN_POINT('Ctrl Pts',(-0.573915184558107,-0.190326085855194,
0.795684265985088));
#10062=CARTESIAN_POINT('Ctrl Pts',(-0.548874290046456,-0.159766064500479,
0.813159949759));
#10063=CARTESIAN_POINT('Ctrl Pts',(-0.537715343527944,-0.142345102874864,
0.820511285096538));
#10064=CARTESIAN_POINT('Ctrl Pts',(-0.517157748491652,-0.0999305678883309,
0.833661031856294));
#10065=CARTESIAN_POINT('Ctrl Pts',(-0.508899795931835,-0.0740444353928835,
0.838633903678357));
#10066=CARTESIAN_POINT('Ctrl Pts',(-0.504455939115716,-0.04763,0.841298510752801));
#10067=CARTESIAN_POINT('Origin',(-0.707106781186548,-0.04763,0.707106781186547));
#10068=CARTESIAN_POINT('Origin',(0.,-0.04763,0.));
#10069=CARTESIAN_POINT('',(-0.951592097314,-0.04763,0.238183666596899));
#10070=CARTESIAN_POINT('Origin',(0.,-0.04763,0.));
#10071=CARTESIAN_POINT('Origin',(-1.,-0.04763,-1.11022302462516E-16));
#10072=CARTESIAN_POINT('Origin',(-1.,0.,-1.11022302462516E-16));
#10073=CARTESIAN_POINT('',(-0.951592097314,-0.04763,-0.2381836665969));
#10074=CARTESIAN_POINT('',(-0.980948,-0.246942143572133,1.08514323328844E-18));
#10075=CARTESIAN_POINT('Ctrl Pts',(-0.951592097314,-0.04763,-0.238183666596899));
#10076=CARTESIAN_POINT('Ctrl Pts',(-0.952850216871763,-0.0740444353928835,
-0.233157223576062));
#10077=CARTESIAN_POINT('Ctrl Pts',(-0.955173119738174,-0.0999305678883309,
-0.223801617934946));
#10078=CARTESIAN_POINT('Ctrl Pts',(-0.960411259488514,-0.142345102874864,
-0.199966927975188));
#10079=CARTESIAN_POINT('Ctrl Pts',(-0.963103647174702,-0.159766064500479,
-0.1868781821531));
#10080=CARTESIAN_POINT('Ctrl Pts',(-0.968453058988463,-0.190326085855194,
-0.15681442133453));
#10081=CARTESIAN_POINT('Ctrl Pts',(-0.971100730005489,-0.203463743702801,
-0.139836317888043));
#10082=CARTESIAN_POINT('Ctrl Pts',(-0.975530745318961,-0.224161999508995,
-0.104422493053067));
#10083=CARTESIAN_POINT('Ctrl Pts',(-0.977553872336861,-0.232861760990032,
-0.0842175114474175));
#10084=CARTESIAN_POINT('Ctrl Pts',(-0.980270995488453,-0.244251601209411,
-0.0421062857595699));
#10085=CARTESIAN_POINT('Ctrl Pts',(-0.980948,-0.246942143572133,-0.0201990724523195));
#10086=CARTESIAN_POINT('Ctrl Pts',(-0.980948,-0.246942143572133,-1.17961196366423E-16));
#10087=CARTESIAN_POINT('Origin',(-1.,-0.04763,-1.11022302462516E-16));
#10088=CARTESIAN_POINT('Ctrl Pts',(-0.980948,-0.246942143572133,-1.17961196366423E-16));
#10089=CARTESIAN_POINT('Ctrl Pts',(-0.980948,-0.246942143572133,0.0201990724523192));
#10090=CARTESIAN_POINT('Ctrl Pts',(-0.980270995488453,-0.244251601209411,
0.0421062857595695));
#10091=CARTESIAN_POINT('Ctrl Pts',(-0.977553872336861,-0.232861760990032,
0.0842175114474169));
#10092=CARTESIAN_POINT('Ctrl Pts',(-0.975530745318961,-0.224161999508995,
0.104422493053066));
#10093=CARTESIAN_POINT('Ctrl Pts',(-0.971100730005489,-0.203463743702801,
0.139836317888042));
#10094=CARTESIAN_POINT('Ctrl Pts',(-0.968453058988463,-0.190326085855194,
0.15681442133453));
#10095=CARTESIAN_POINT('Ctrl Pts',(-0.963103647174702,-0.15976606450048,
0.1868781821531));
#10096=CARTESIAN_POINT('Ctrl Pts',(-0.960411259488514,-0.142345102874864,
0.199966927975188));
#10097=CARTESIAN_POINT('Ctrl Pts',(-0.955173119738174,-0.099930567888331,
0.223801617934945));
#10098=CARTESIAN_POINT('Ctrl Pts',(-0.952850216871763,-0.0740444353928835,
0.233157223576061));
#10099=CARTESIAN_POINT('Ctrl Pts',(-0.951592097314,-0.04763,0.238183666596899));
#10100=CARTESIAN_POINT('Origin',(0.,-0.04763,0.));
#10101=CARTESIAN_POINT('',(-0.841298510752802,-0.04763,-0.504455939115715));
#10102=CARTESIAN_POINT('Origin',(0.,-0.04763,0.));
#10103=CARTESIAN_POINT('Origin',(-0.707106781186547,-0.04763,-0.707106781186548));
#10104=CARTESIAN_POINT('Origin',(-0.707106781186547,0.,-0.707106781186548));
#10105=CARTESIAN_POINT('',(-0.504455939115715,-0.04763,-0.841298510752802));
#10106=CARTESIAN_POINT('Ctrl Pts',(-0.504455939115715,-0.04763,-0.841298510752802));
#10107=CARTESIAN_POINT('Ctrl Pts',(-0.508899795931835,-0.0740444353928835,
-0.838633903678357));
#10108=CARTESIAN_POINT('Ctrl Pts',(-0.517157748491652,-0.0999305678883309,
-0.833661031856294));
#10109=CARTESIAN_POINT('Ctrl Pts',(-0.537715343527944,-0.142345102874864,
-0.820511285096538));
#10110=CARTESIAN_POINT('Ctrl Pts',(-0.548874290046456,-0.159766064500479,
-0.813159949759));
#10111=CARTESIAN_POINT('Ctrl Pts',(-0.573915184558107,-0.190326085855194,
-0.795684265985089));
#10112=CARTESIAN_POINT('Ctrl Pts',(-0.587792702767295,-0.203463743702801,
-0.78555112003688));
#10113=CARTESIAN_POINT('Ctrl Pts',(-0.615966552324775,-0.224161999508995,
-0.763642258217233));
#10114=CARTESIAN_POINT('Ctrl Pts',(-0.631684198665438,-0.232861760990032,
-0.750785745543687));
#10115=CARTESIAN_POINT('Ctrl Pts',(-0.663382628119203,-0.244251601209411,
-0.722929908501543));
#10116=CARTESIAN_POINT('Ctrl Pts',(-0.679352081686668,-0.246942143572133,
-0.707917883896095));
#10117=CARTESIAN_POINT('Ctrl Pts',(-0.707917883896095,-0.246942143572133,
-0.679352081686668));
#10118=CARTESIAN_POINT('Ctrl Pts',(-0.722929908501543,-0.244251601209411,
-0.663382628119203));
#10119=CARTESIAN_POINT('Ctrl Pts',(-0.750785745543687,-0.232861760990032,
-0.631684198665439));
#10120=CARTESIAN_POINT('Ctrl Pts',(-0.763642258217232,-0.224161999508995,
-0.615966552324775));
#10121=CARTESIAN_POINT('Ctrl Pts',(-0.78555112003688,-0.203463743702801,
-0.587792702767295));
#10122=CARTESIAN_POINT('Ctrl Pts',(-0.795684265985088,-0.190326085855194,
-0.573915184558107));
#10123=CARTESIAN_POINT('Ctrl Pts',(-0.813159949759,-0.15976606450048,-0.548874290046456));
#10124=CARTESIAN_POINT('Ctrl Pts',(-0.820511285096538,-0.142345102874864,
-0.537715343527944));
#10125=CARTESIAN_POINT('Ctrl Pts',(-0.833661031856294,-0.0999305678883311,
-0.517157748491652));
#10126=CARTESIAN_POINT('Ctrl Pts',(-0.838633903678357,-0.0740444353928836,
-0.508899795931835));
#10127=CARTESIAN_POINT('Ctrl Pts',(-0.841298510752801,-0.04763,-0.504455939115715));
#10128=CARTESIAN_POINT('Origin',(-0.707106781186547,-0.04763,-0.707106781186548));
#10129=CARTESIAN_POINT('Origin',(0.,-0.04763,0.));
#10130=CARTESIAN_POINT('',(-0.238183666596899,-0.04763,-0.951592097314));
#10131=CARTESIAN_POINT('Origin',(0.,-0.04763,0.));
#10132=CARTESIAN_POINT('Origin',(5.55111512312578E-17,-0.04763,-1.));
#10133=CARTESIAN_POINT('Origin',(5.55111512312578E-17,0.,-1.));
#10134=CARTESIAN_POINT('',(0.238183666596899,-0.04763,-0.951592097314));
#10135=CARTESIAN_POINT('Ctrl Pts',(0.238183666596899,-0.04763,-0.951592097314));
#10136=CARTESIAN_POINT('Ctrl Pts',(0.233157223576062,-0.0740444353928835,
-0.952850216871763));
#10137=CARTESIAN_POINT('Ctrl Pts',(0.223801617934946,-0.099930567888331,
-0.955173119738174));
#10138=CARTESIAN_POINT('Ctrl Pts',(0.199966927975188,-0.142345102874864,
-0.960411259488514));
#10139=CARTESIAN_POINT('Ctrl Pts',(0.1868781821531,-0.15976606450048,-0.963103647174702));
#10140=CARTESIAN_POINT('Ctrl Pts',(0.15681442133453,-0.190326085855194,
-0.968453058988463));
#10141=CARTESIAN_POINT('Ctrl Pts',(0.139836317888042,-0.203463743702801,
-0.971100730005489));
#10142=CARTESIAN_POINT('Ctrl Pts',(0.104422493053067,-0.224161999508995,
-0.975530745318961));
#10143=CARTESIAN_POINT('Ctrl Pts',(0.0842175114474173,-0.232861760990032,
-0.977553872336861));
#10144=CARTESIAN_POINT('Ctrl Pts',(0.0421062857595698,-0.244251601209411,
-0.980270995488453));
#10145=CARTESIAN_POINT('Ctrl Pts',(0.0201990724523194,-0.246942143572133,
-0.980948));
#10146=CARTESIAN_POINT('Ctrl Pts',(-0.0201990724523193,-0.246942143572133,
-0.980948));
#10147=CARTESIAN_POINT('Ctrl Pts',(-0.0421062857595697,-0.244251601209411,
-0.980270995488453));
#10148=CARTESIAN_POINT('Ctrl Pts',(-0.0842175114474171,-0.232861760990032,
-0.977553872336861));
#10149=CARTESIAN_POINT('Ctrl Pts',(-0.104422493053067,-0.224161999508995,
-0.975530745318961));
#10150=CARTESIAN_POINT('Ctrl Pts',(-0.139836317888042,-0.203463743702801,
-0.971100730005489));
#10151=CARTESIAN_POINT('Ctrl Pts',(-0.15681442133453,-0.190326085855194,
-0.968453058988463));
#10152=CARTESIAN_POINT('Ctrl Pts',(-0.1868781821531,-0.15976606450048,-0.963103647174702));
#10153=CARTESIAN_POINT('Ctrl Pts',(-0.199966927975188,-0.142345102874864,
-0.960411259488514));
#10154=CARTESIAN_POINT('Ctrl Pts',(-0.223801617934945,-0.099930567888331,
-0.955173119738174));
#10155=CARTESIAN_POINT('Ctrl Pts',(-0.233157223576062,-0.0740444353928835,
-0.952850216871763));
#10156=CARTESIAN_POINT('Ctrl Pts',(-0.238183666596899,-0.0476299999999999,
-0.951592097314));
#10157=CARTESIAN_POINT('Origin',(5.55111512312578E-17,-0.04763,-1.));
#10158=CARTESIAN_POINT('Origin',(0.,-0.04763,0.));
#10159=CARTESIAN_POINT('',(0.504455939115715,-0.04763,-0.841298510752802));
#10160=CARTESIAN_POINT('Origin',(0.,-0.04763,0.));
#10161=CARTESIAN_POINT('Origin',(0.707106781186548,-0.04763,-0.707106781186547));
#10162=CARTESIAN_POINT('Origin',(0.707106781186548,0.,-0.707106781186547));
#10163=CARTESIAN_POINT('',(0.841298510752802,-0.04763,-0.504455939115715));
#10164=CARTESIAN_POINT('Ctrl Pts',(0.841298510752802,-0.04763,-0.504455939115715));
#10165=CARTESIAN_POINT('Ctrl Pts',(0.838633903678357,-0.0740444353928835,
-0.508899795931835));
#10166=CARTESIAN_POINT('Ctrl Pts',(0.833661031856294,-0.0999305678883309,
-0.517157748491652));
#10167=CARTESIAN_POINT('Ctrl Pts',(0.820511285096538,-0.142345102874864,
-0.537715343527944));
#10168=CARTESIAN_POINT('Ctrl Pts',(0.813159949759,-0.159766064500479,-0.548874290046456));
#10169=CARTESIAN_POINT('Ctrl Pts',(0.795684265985088,-0.190326085855194,
-0.573915184558107));
#10170=CARTESIAN_POINT('Ctrl Pts',(0.78555112003688,-0.203463743702801,
-0.587792702767295));
#10171=CARTESIAN_POINT('Ctrl Pts',(0.763642258217233,-0.224161999508995,
-0.615966552324775));
#10172=CARTESIAN_POINT('Ctrl Pts',(0.750785745543687,-0.232861760990032,
-0.631684198665438));
#10173=CARTESIAN_POINT('Ctrl Pts',(0.722929908501543,-0.244251601209411,
-0.663382628119203));
#10174=CARTESIAN_POINT('Ctrl Pts',(0.707917883896095,-0.246942143572133,
-0.679352081686668));
#10175=CARTESIAN_POINT('Ctrl Pts',(0.679352081686668,-0.246942143572133,
-0.707917883896095));
#10176=CARTESIAN_POINT('Ctrl Pts',(0.663382628119203,-0.244251601209411,
-0.722929908501543));
#10177=CARTESIAN_POINT('Ctrl Pts',(0.631684198665438,-0.232861760990032,
-0.750785745543687));
#10178=CARTESIAN_POINT('Ctrl Pts',(0.615966552324775,-0.224161999508995,
-0.763642258217232));
#10179=CARTESIAN_POINT('Ctrl Pts',(0.587792702767295,-0.203463743702801,
-0.78555112003688));
#10180=CARTESIAN_POINT('Ctrl Pts',(0.573915184558107,-0.190326085855194,
-0.795684265985088));
#10181=CARTESIAN_POINT('Ctrl Pts',(0.548874290046456,-0.159766064500479,
-0.813159949759));
#10182=CARTESIAN_POINT('Ctrl Pts',(0.537715343527944,-0.142345102874864,
-0.820511285096538));
#10183=CARTESIAN_POINT('Ctrl Pts',(0.517157748491652,-0.099930567888331,
-0.833661031856294));
#10184=CARTESIAN_POINT('Ctrl Pts',(0.508899795931835,-0.0740444353928835,
-0.838633903678357));
#10185=CARTESIAN_POINT('Ctrl Pts',(0.504455939115715,-0.04763,-0.841298510752801));
#10186=CARTESIAN_POINT('Origin',(0.707106781186548,-0.04763,-0.707106781186547));
#10187=CARTESIAN_POINT('Origin',(0.,-0.166705,0.));
#10188=CARTESIAN_POINT('',(-0.980948,-0.28578,1.20131482833E-16));
#10189=CARTESIAN_POINT('Origin',(0.,-0.28578,0.));
#10190=CARTESIAN_POINT('',(-0.980948,-0.166705,1.20131482833E-16));
#10191=CARTESIAN_POINT('',(0.951592097314,-0.04763,0.238183666596899));
#10192=CARTESIAN_POINT('Origin',(0.,-0.04763,0.));
#10193=CARTESIAN_POINT('',(0.951592097314,-0.04763,-0.238183666596899));
#10194=CARTESIAN_POINT('Ctrl Pts',(0.951592097314,-0.04763,0.238183666596899));
#10195=CARTESIAN_POINT('Ctrl Pts',(0.952850216871763,-0.0740444353928835,
0.233157223576062));
#10196=CARTESIAN_POINT('Ctrl Pts',(0.955173119738174,-0.099930567888331,
0.223801617934945));
#10197=CARTESIAN_POINT('Ctrl Pts',(0.960411259488514,-0.142345102874864,
0.199966927975188));
#10198=CARTESIAN_POINT('Ctrl Pts',(0.963103647174702,-0.15976606450048,
0.1868781821531));
#10199=CARTESIAN_POINT('Ctrl Pts',(0.968453058988463,-0.190326085855194,
0.15681442133453));
#10200=CARTESIAN_POINT('Ctrl Pts',(0.971100730005489,-0.203463743702801,
0.139836317888042));
#10201=CARTESIAN_POINT('Ctrl Pts',(0.975530745318961,-0.224161999508995,
0.104422493053067));
#10202=CARTESIAN_POINT('Ctrl Pts',(0.977553872336861,-0.232861760990032,
0.0842175114474172));
#10203=CARTESIAN_POINT('Ctrl Pts',(0.980270995488453,-0.244251601209411,
0.0421062857595697));
#10204=CARTESIAN_POINT('Ctrl Pts',(0.980948,-0.246942143572133,0.0201990724523194));
#10205=CARTESIAN_POINT('Ctrl Pts',(0.980948,-0.246942143572133,-0.0201990724523194));
#10206=CARTESIAN_POINT('Ctrl Pts',(0.980270995488453,-0.244251601209411,
-0.0421062857595697));
#10207=CARTESIAN_POINT('Ctrl Pts',(0.977553872336861,-0.232861760990032,
-0.0842175114474172));
#10208=CARTESIAN_POINT('Ctrl Pts',(0.975530745318961,-0.224161999508995,
-0.104422493053067));
#10209=CARTESIAN_POINT('Ctrl Pts',(0.971100730005489,-0.203463743702801,
-0.139836317888042));
#10210=CARTESIAN_POINT('Ctrl Pts',(0.968453058988463,-0.190326085855194,
-0.15681442133453));
#10211=CARTESIAN_POINT('Ctrl Pts',(0.963103647174702,-0.15976606450048,
-0.1868781821531));
#10212=CARTESIAN_POINT('Ctrl Pts',(0.960411259488514,-0.142345102874864,
-0.199966927975188));
#10213=CARTESIAN_POINT('Ctrl Pts',(0.955173119738174,-0.099930567888331,
-0.223801617934945));
#10214=CARTESIAN_POINT('Ctrl Pts',(0.952850216871763,-0.0740444353928835,
-0.233157223576062));
#10215=CARTESIAN_POINT('Ctrl Pts',(0.951592097314,-0.0476299999999999,-0.238183666596899));
#10216=CARTESIAN_POINT('Origin',(0.,-0.04763,0.));
#10217=CARTESIAN_POINT('Origin',(0.,-0.04763,0.));
#10218=CARTESIAN_POINT('Origin',(1.,-0.04763,0.));
#10219=CARTESIAN_POINT('Origin',(1.,0.,0.));
#10220=CARTESIAN_POINT('Origin',(1.,-0.04763,0.));
#10221=CARTESIAN_POINT('Origin',(0.,-0.28578,0.));
#10222=CARTESIAN_POINT('Origin',(0.,-0.04763,0.));
#10585=UNCERTAINTY_MEASURE_WITH_UNIT(LENGTH_MEASURE(0.001),#10628,
'DISTANCE_ACCURACY_VALUE',
'Maximum model space distance between geometric entities at asserted c
onnectivities');
#10595=UNCERTAINTY_MEASURE_WITH_UNIT(LENGTH_MEASURE(0.001),#10628,
'DISTANCE_ACCURACY_VALUE',
'Maximum model space distance between geometric entities at asserted c
onnectivities');
#10617=(
GEOMETRIC_REPRESENTATION_CONTEXT(3)
GLOBAL_UNCERTAINTY_ASSIGNED_CONTEXT((#10585))
GLOBAL_UNIT_ASSIGNED_CONTEXT((#10628,#10630,#10631))
REPRESENTATION_CONTEXT('','3D')
);
#10627=(
GEOMETRIC_REPRESENTATION_CONTEXT(3)
GLOBAL_UNCERTAINTY_ASSIGNED_CONTEXT((#10595))
GLOBAL_UNIT_ASSIGNED_CONTEXT((#10628,#10630,#10631))
REPRESENTATION_CONTEXT('','3D')
);
#10628=(
LENGTH_UNIT()
NAMED_UNIT(*)
SI_UNIT(.CENTI.,.METRE.)
);
#10630=(
NAMED_UNIT(*)
PLANE_ANGLE_UNIT()
SI_UNIT($,.RADIAN.)
);
#10631=(
NAMED_UNIT(*)
SI_UNIT($,.STERADIAN.)
SOLID_ANGLE_UNIT()
);
#10653=SHAPE_DEFINITION_REPRESENTATION(#10694,#10758);
#10694=PRODUCT_DEFINITION_SHAPE('',$,#10790);
#10758=SHAPE_REPRESENTATION('',(#5637),#10617);
#10768=PRODUCT_DEFINITION_CONTEXT('part definition',#10863,'design');
#10790=PRODUCT_DEFINITION('Cage','Cage',#10821,#10768);
#10821=PRODUCT_DEFINITION_FORMATION('',$,#10886);
#10863=APPLICATION_CONTEXT(
'Core Data for Automotive Mechanical Design Process');
#10864=PRODUCT_CONTEXT('part definition',#10863,'mechanical');
#10886=PRODUCT('Cage','Cage','Cage',(#10864));
#10959=COLOUR_RGB('Grey',0.48,0.52,0.57);
#10960=FILL_AREA_STYLE_COLOUR('',#10959);
#10961=FILL_AREA_STYLE('',(#10960));
#10962=SURFACE_STYLE_FILL_AREA(#10961);
#10963=SURFACE_SIDE_STYLE('',(#10962));
#10964=SURFACE_STYLE_USAGE(.BOTH.,#10963);
#10965=PRESENTATION_STYLE_ASSIGNMENT((#10964));
ENDSEC;
END-ISO-10303-21;
